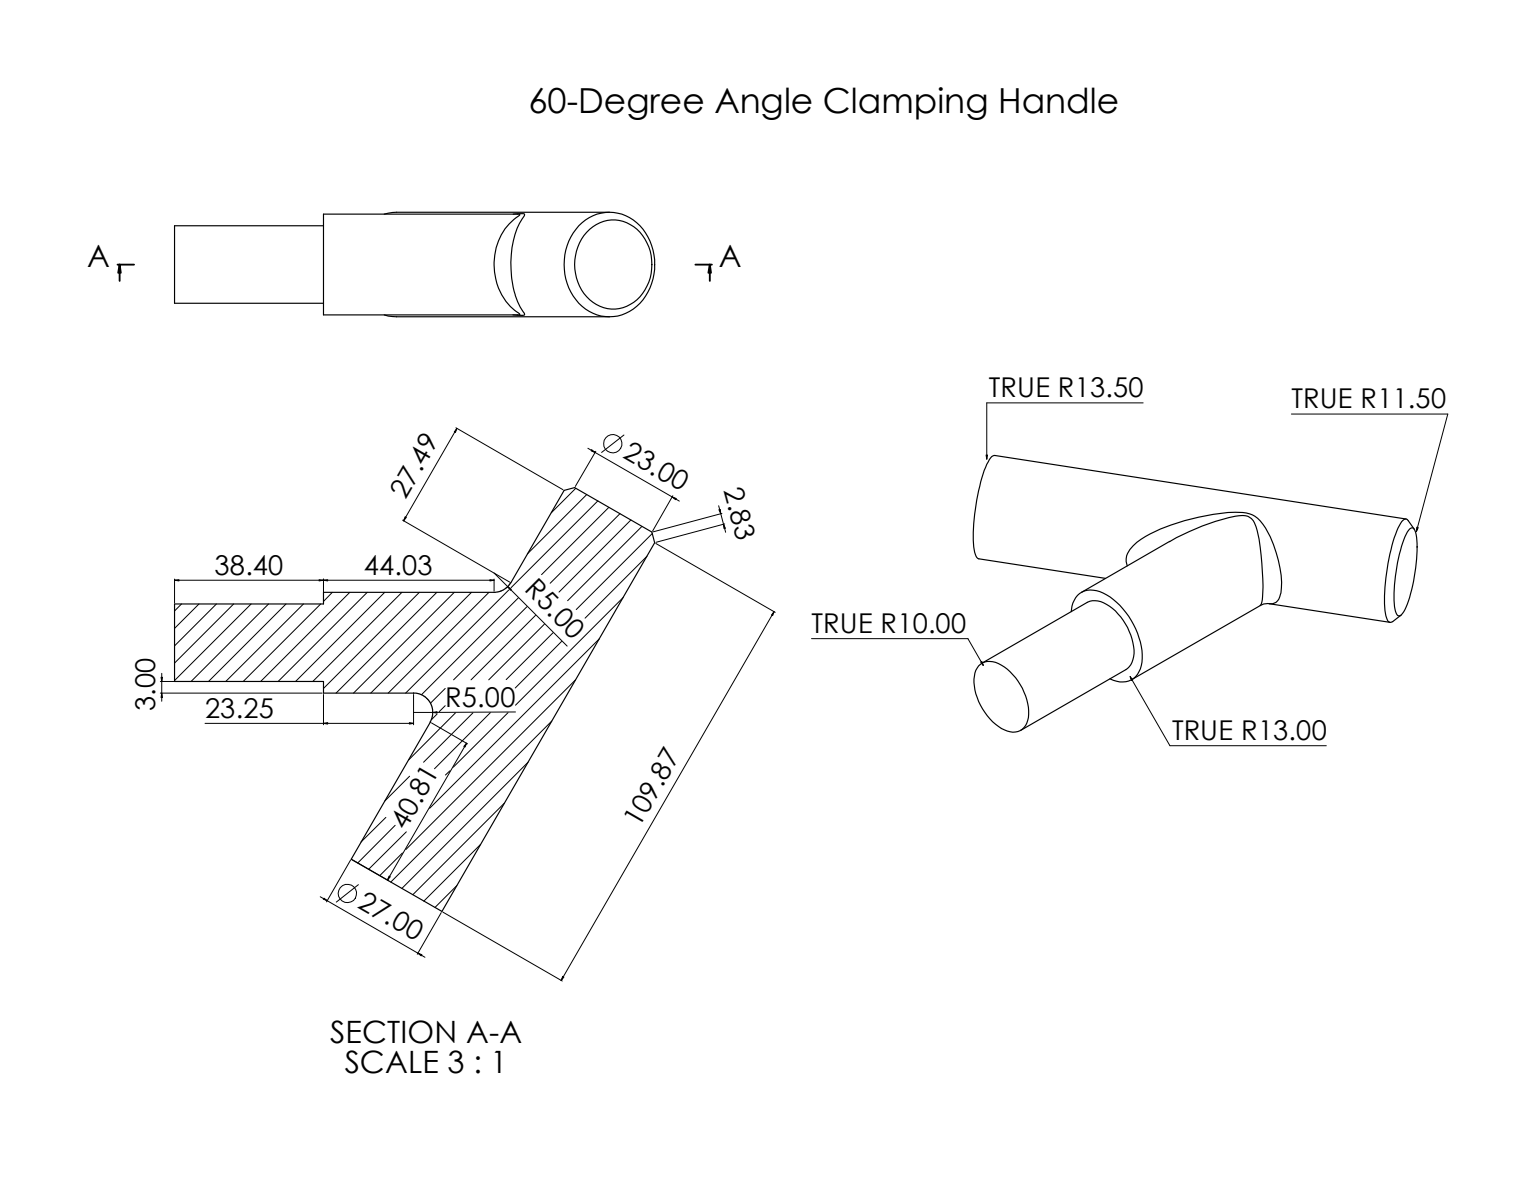
ISO-10303-21;
HEADER;
FILE_DESCRIPTION (('STEP AP214'),
    '1' );
FILE_NAME ('60-Degree Angle Clamping Handle.step',
    '2026-10-26T22:46:44',
    ( '' ),
    ( '' ),
    'SwSTEP 2.0',
    'SolidWorks 2025',
    '' );
FILE_SCHEMA (( 'AUTOMOTIVE_DESIGN' ));
ENDSEC;

DATA;
#3=CARTESIAN_POINT ( 'NONE',  ( 65.59213978856993776, 73.13321318536134186, -22.65145034150330616 ) ) ;
#7=CARTESIAN_POINT ( 'NONE',  ( 63.07699891084844523, 77.89006876494195808, -8.475025019650114899 ) ) ;
#33=CARTESIAN_POINT ( 'NONE',  ( 72.20123527641440830, 74.90140838070377072, -0.9291223156572469000 ) ) ;
#36=EDGE_CURVE ( 'NONE', #14580, #7029, #1544, .T. ) ;
#50=CARTESIAN_POINT ( 'NONE',  ( 54.22345804136912051, 78.00945976696758066, -12.46744236580036791 ) ) ;
#59=AXIS2_PLACEMENT_3D ( 'NONE', #20205, #816, #18936 ) ;
#61=EDGE_CURVE ( 'NONE', #19064, #20850, #19152, .T. ) ;
#66=B_SPLINE_CURVE_WITH_KNOTS ( 'NONE', 3,
 ( #8841, #10417, #10308, #18497, #16902, #3750, #6925, #16700, #20081, #8735, #685, #15341, #16481, #1963, #8630, #5225, #15026, #3643, #15129, #584, #2382, #3544, #11613, #795, #7034, #9988, #7140, #8411, #10096, #5431, #7246, #2073, #5545, #13520, #19652, #19965, #12034, #14912, #20596, #12135, #15751, #14164, #15438, #7666 ),
 .UNSPECIFIED., .F., .F.,
 ( 4, 2, 2, 2, 2, 2, 2, 2, 2, 2, 2, 2, 2, 2, 2, 2, 2, 2, 2, 2, 2, 4 ),
 ( 0.09617483233575800650, 0.09914136407045009980, 0.1006246299377961534, 0.1021078958051422070, 0.1050744275398343142, 0.1080409592745264352, 0.1095242251418725027, 0.1110074910092185702, 0.1139740227439106635, 0.1154572886112567032, 0.1169405544786027568, 0.1176821874122757766, 0.1184238203459488104, 0.1199070862132948084, 0.1213903520806408065, 0.1228736179479868185, 0.1258401496826788146, 0.1288066814173708385, 0.1317732131520628625, 0.1377062766214468548, 0.1406728083561389064, 0.1436393400908309581 ),
 .UNSPECIFIED. ) ;
#114=CARTESIAN_POINT ( 'NONE',  ( 60.67510459333478678, 75.25732190833497270, -4.504626686252581891 ) ) ;
#134=CARTESIAN_POINT ( 'NONE',  ( 79.71489363099678371, 68.48589378271981332, 0.4850882486192328313 ) ) ;
#137=CARTESIAN_POINT ( 'NONE',  ( 78.24291704612552678, 52.61578353862905288, -16.49051273642769289 ) ) ;
#149=CARTESIAN_POINT ( 'NONE',  ( 55.21771490548105987, 77.58705400462579860, -9.223793769219156502 ) ) ;
#167=CARTESIAN_POINT ( 'NONE',  ( 64.57205371728791476, 77.00255147951500589, -18.47244162738281048 ) ) ;
#187=CARTESIAN_POINT ( 'NONE',  ( 31.00000000000000711, 65.00000000000000000, 0.4999999999999970024 ) ) ;
#188=CARTESIAN_POINT ( 'NONE',  ( 61.55523633728010680, 134.3395726428436774, -12.50000000000000000 ) ) ;
#207=CARTESIAN_POINT ( 'NONE',  ( 54.88115708448756891, 77.73008567377026168, -9.852707893755395574 ) ) ;
#225=CARTESIAN_POINT ( 'NONE',  ( 58.57586221349340860, 85.49999999999941735, -12.75852093573072032 ) ) ;
#232=ORIENTED_EDGE ( 'NONE', *, *, #19491, .T. ) ;
#235=CARTESIAN_POINT ( 'NONE',  ( 82.91273300024698756, 62.96352848655696732, 0.4857625843512909936 ) ) ;
#237=CARTESIAN_POINT ( 'NONE',  ( 79.37077236198800279, 49.52807498578272316, -11.55216451523023657 ) ) ;
#250=CARTESIAN_POINT ( 'NONE',  ( 69.27805541368826425, 71.51676853726520733, -1.217222206000668994 ) ) ;
#268=CARTESIAN_POINT ( 'NONE',  ( 79.94330251453826008, 67.07585766759784462, -25.35419664930641659 ) ) ;
#308=CARTESIAN_POINT ( 'NONE',  ( 57.74218117268578965, 76.51201622986452833, -6.446212979376384489 ) ) ;
#332=VECTOR ( 'NONE', #6843, 1000.000000000000114 ) ;
#342=CARTESIAN_POINT ( 'NONE',  ( 76.94659547200038219, 54.56764967722406823, -20.27289619944112786 ) ) ;
#354=CARTESIAN_POINT ( 'NONE',  ( 76.60035650392514128, 54.09786888454211606, -5.411621923353880703 ) ) ;
#364=CARTESIAN_POINT ( 'NONE',  ( 54.28616200159638083, 77.98283342922744055, -13.21260929400889950 ) ) ;
#383=CARTESIAN_POINT ( 'NONE',  ( 81.91557740337785276, 60.53556548035048479, -24.72568746032316511 ) ) ;
#424=CARTESIAN_POINT ( 'NONE',  ( 64.92628429094538944, 80.60227088397526529, -21.04771496906974804 ) ) ;
#444=CARTESIAN_POINT ( 'NONE',  ( 116.4887320753796587, 39.19196698708793747, -12.50000000000000000 ) ) ;
#452=CARTESIAN_POINT ( 'NONE',  ( 77.98814704359870120, 52.13394603002385708, -14.43366844821333572 ) ) ;
#460=CARTESIAN_POINT ( 'NONE',  ( 76.86601529753625073, 54.45829969532270809, -4.885926103426701417 ) ) ;
#468=CARTESIAN_POINT ( 'NONE',  ( 58.42188568717646291, 76.22201287237797374, -19.09002448919735428 ) ) ;
#490=EDGE_CURVE ( 'NONE', #14308, #10603, #66, .T. ) ;
#492=CARTESIAN_POINT ( 'NONE',  ( 82.72938175528729232, 60.17526287326926848, -24.94610863806802925 ) ) ;
#510=CARTESIAN_POINT ( 'NONE',  ( 78.47145885649602803, 56.68941013563004816, -2.495457786690434610 ) ) ;
#516=EDGE_LOOP ( 'NONE', ( #16773, #17609, #13168, #2183, #18368 ) ) ;
#526=CARTESIAN_POINT ( 'NONE',  ( 54.80454468582367866, 77.76263990853003349, -14.98572519218623889 ) ) ;
#549=CARTESIAN_POINT ( 'NONE',  ( 82.83076346201933404, 60.85614612423834302, 0.1131946898860237832 ) ) ;
#551=CARTESIAN_POINT ( 'NONE',  ( 79.48072094348276551, 49.82842808374601162, -15.22942965609466270 ) ) ;
#584=CARTESIAN_POINT ( 'NONE',  ( 82.93056326137615031, 61.76632323605970498, -25.30877389655469756 ) ) ;
#588=CARTESIAN_POINT ( 'NONE',  ( 81.35624441458497813, 64.60845994063853936, -25.49655522582468237 ) ) ;
#594=CARTESIAN_POINT ( 'NONE',  ( 86.00000000000000000, 65.00000000000000000, -12.50000000000000000 ) ) ;
#609=CARTESIAN_POINT ( 'NONE',  ( 78.05328906524978549, 56.09831538232894843, -3.025823995327162841 ) ) ;
#628=CARTESIAN_POINT ( 'NONE',  ( 55.63769925775388714, 77.40847683933932899, -16.40349017008347587 ) ) ;
#651=CARTESIAN_POINT ( 'NONE',  ( 79.92501236954103661, 58.85901869437554268, -1.031643761997860897 ) ) ;
#660=CARTESIAN_POINT ( 'NONE',  ( 75.12482142704125465, 52.12498453794043485, -14.42445013263158238 ) ) ;
#685=CARTESIAN_POINT ( 'NONE',  ( 80.96866787924291486, 54.01966784746423400, -21.77093191989936471 ) ) ;
#687=DIRECTION ( 'NONE',  ( 0.8660254037844362651, 0.5000000000000043299, 0.000000000000000000 ) ) ;
#690=CARTESIAN_POINT ( 'NONE',  ( 80.82058163573867660, 65.29640235792498970, -25.49857619709358048 ) ) ;
#692=CARTESIAN_POINT ( 'NONE',  ( 59.45914026090133575, 84.82127241994479050, -15.89427485249682626 ) ) ;
#713=CARTESIAN_POINT ( 'NONE',  ( 79.12402306321216372, 57.63706906876117131, -1.778930141804763831 ) ) ;
#735=CARTESIAN_POINT ( 'NONE',  ( 60.75134160315762699, 83.82709006120157369, -17.71883169751006548 ) ) ;
#765=CARTESIAN_POINT ( 'NONE',  ( 81.28584910398754459, 61.36302568043885941, -0.01657068726255144647 ) ) ;
#773=CARTESIAN_POINT ( 'NONE',  ( 78.91362683933590461, 57.32445438350235634, -23.00962568793631036 ) ) ;
#779=MECHANICAL_DESIGN_GEOMETRIC_PRESENTATION_REPRESENTATION('',(#4502),#19384);
#795=CARTESIAN_POINT ( 'NONE',  ( 82.80106909841869367, 63.71549435008554241, -25.56184987062727743 ) ) ;
#800=CARTESIAN_POINT ( 'NONE',  ( 81.32899831459523909, 65.64633111285905898, -25.49135248455479541 ) ) ;
#816=DIRECTION ( 'NONE',  ( 1.000000000000000000, -0.000000000000000000, -0.000000000000000000 ) ) ;
#838=CARTESIAN_POINT ( 'NONE',  ( 63.10828723790488937, 82.00971617295591898, -19.89823807612492601 ) ) ;
#863=CARTESIAN_POINT ( 'NONE',  ( 81.25108741995337880, 54.86839436850289076, -2.588578014267536975 ) ) ;
#875=FACE_BOUND ( 'NONE', #4618, .T. ) ;
#955=DIRECTION ( 'NONE',  ( 0.5705585702127619063, 0.000000000000000000, 0.8212569134910030488 ) ) ;
#957=CARTESIAN_POINT ( 'NONE',  ( -7.400583024429460366, 65.00000000000000000, -12.50000000000000000 ) ) ;
#967=CARTESIAN_POINT ( 'NONE',  ( 80.52543256968870367, 57.14253470624510811, -2.115012055466068741 ) ) ;
#969=ORIENTED_EDGE ( 'NONE', *, *, #20916, .T. ) ;
#973=CARTESIAN_POINT ( 'NONE',  ( 79.14338724215045318, 54.34411555289009499, -5.006392671230091906 ) ) ;
#991=PLANE ( 'NONE',  #9815 ) ;
#1001=AXIS2_PLACEMENT_3D ( 'NONE', #3701, #10052, #11562 ) ;
#1027=CARTESIAN_POINT ( 'NONE',  ( 80.02281011973705915, 51.32424184041445159, -6.278812083988356996 ) ) ;
#1031=CONICAL_SURFACE ( 'NONE', #12883, 11.50000000000002309, 0.7853981633974477239 ) ;
#1052=ORIENTED_EDGE ( 'NONE', *, *, #9633, .T. ) ;
#1077=CARTESIAN_POINT ( 'NONE',  ( 75.33430881385784517, 70.41445892100490767, -0.5834797149646978598 ) ) ;
#1137=ORIENTED_EDGE ( 'NONE', *, *, #36, .F. ) ;
#1182=CARTESIAN_POINT ( 'NONE',  ( 76.96076175570429712, 69.31984913612060950, -0.1862401116020122038 ) ) ;
#1202=DIRECTION ( 'NONE',  ( -0.5000000000000045519, 0.8660254037844360431, 0.000000000000000000 ) ) ;
#1274=DIRECTION ( 'NONE',  ( 0.000000000000000000, 0.000000000000000000, 1.000000000000000000 ) ) ;
#1289=CARTESIAN_POINT ( 'NONE',  ( 71.98518577010987940, 75.06736630765306018, -1.005590943479974131 ) ) ;
#1309=CARTESIAN_POINT ( 'NONE',  ( -7.400583024429460366, 65.00000000000000000, -2.500000000000005773 ) ) ;
#1379=CARTESIAN_POINT ( 'NONE',  ( 61.57468973143931379, 74.87077495648827608, -20.95977551465544764 ) ) ;
#1387=CARTESIAN_POINT ( 'NONE',  ( 77.64194032647326082, 70.38417867298623776, 0.2137292797775141029 ) ) ;
#1409=EDGE_CURVE ( 'NONE', #2714, #10603, #16734, .T. ) ;
#1417=CARTESIAN_POINT ( 'NONE',  ( 58.59049733147158889, 85.48875911470162237, -11.99710087975904216 ) ) ;
#1456=CARTESIAN_POINT ( 'NONE',  ( 64.92628429094538944, 80.60227088397526529, -21.04771496906974448 ) ) ;
#1490=CARTESIAN_POINT ( 'NONE',  ( 82.46725602463313010, 64.79916592910645079, 0.6251661754290179784 ) ) ;
#1503=CARTESIAN_POINT ( 'NONE',  ( 86.00000000000000000, 65.00000000000000000, -12.50000000000000000 ) ) ;
#1518=CARTESIAN_POINT ( 'NONE',  ( 82.69314351557979137, 60.01919287894784105, -0.1021492064584022391 ) ) ;
#1544=CIRCLE ( 'NONE', #20817, 13.49999999999999645 ) ;
#1586=CARTESIAN_POINT ( 'NONE',  ( 68.05653244943854929, 72.05492144323341108, -23.45593384645862045 ) ) ;
#1591=PLANE ( 'NONE',  #12909 ) ;
#1595=CARTESIAN_POINT ( 'NONE',  ( 60.86250686525652753, 83.74154639049930893, -7.143441593098562414 ) ) ;
#1638=CARTESIAN_POINT ( 'NONE',  ( 79.60954748500523692, 66.31227659742221192, 0.4370474645863004493 ) ) ;
#1657=CARTESIAN_POINT ( 'NONE',  ( 75.15087072258846490, 70.53326157795075346, -24.36499220651786146 ) ) ;
#1659=CIRCLE ( 'NONE', #19280, 9.999999999999994671 ) ;
#1661=CARTESIAN_POINT ( 'NONE',  ( 105.7973891242897650, 30.70991617951901276, -12.50000000000000000 ) ) ;
#1694=CARTESIAN_POINT ( 'NONE',  ( 55.27961512323265225, 77.56072257029609318, -9.140361019020206257 ) ) ;
#1706=CARTESIAN_POINT ( 'NONE',  ( 31.00000000000000711, 65.00000000000000000, -12.50000000000000000 ) ) ;
#1719=CARTESIAN_POINT ( 'NONE',  ( 82.78189083499628964, 60.49709294355461253, 0.02860270449327129150 ) ) ;
#1725=CARTESIAN_POINT ( 'NONE',  ( 77.91922477836661187, 52.00401066416952034, -13.06454345700202424 ) ) ;
#1742=CARTESIAN_POINT ( 'NONE',  ( 57.02843452872113517, 76.81644352065700332, -7.029764943285477408 ) ) ;
#1762=CARTESIAN_POINT ( 'NONE',  ( 76.57684527313351452, 68.08025284203007743, -25.13374168853553670 ) ) ;
#1764=ADVANCED_FACE ( 'NONE', ( #10312 ), #15343, .T. ) ;
#1804=CARTESIAN_POINT ( 'NONE',  ( 62.19571619003149010, 78.41436756500478111, -11.69768420993622904 ) ) ;
#1824=CARTESIAN_POINT ( 'NONE',  ( 78.98475196968189493, 69.17512925677146995, 0.4016226566437379741 ) ) ;
#1829=CARTESIAN_POINT ( 'NONE',  ( 75.20419437876392976, 52.23006250689047647, -10.01053177166429542 ) ) ;
#1847=CARTESIAN_POINT ( 'NONE',  ( 56.65135822015081146, 76.97701555849656074, -17.56718000666989354 ) ) ;
#1865=CARTESIAN_POINT ( 'NONE',  ( 78.39368881307802894, 68.30389099123098617, -25.10803604556682700 ) ) ;
#1905=ORIENTED_EDGE ( 'NONE', *, *, #2268, .T. ) ;
#1908=CARTESIAN_POINT ( 'NONE',  ( 62.82311980245329153, 82.22968959821695023, -5.348578013552717003 ) ) ;
#1936=CARTESIAN_POINT ( 'NONE',  ( 79.67147709189563898, 50.35212617480907227, -8.215081154367272376 ) ) ;
#1940=ORIENTED_EDGE ( 'NONE', *, *, #10019, .F. ) ;
#1950=CARTESIAN_POINT ( 'NONE',  ( 71.88466637961029448, 70.33575297470315491, -0.6373663580885260416 ) ) ;
#1951=VECTOR ( 'NONE', #13576, 1000.000000000000000 ) ;
#1961=DIRECTION ( 'NONE',  ( 1.000000000000000000, -0.000000000000000000, -0.000000000000000000 ) ) ;
#1963=CARTESIAN_POINT ( 'NONE',  ( 81.73016281821475104, 56.36132269136237483, -23.36898426428367870 ) ) ;
#1969=CARTESIAN_POINT ( 'NONE',  ( 68.88680438096986336, 74.41951537632650115, -21.80366467887538917 ) ) ;
#1975=DIRECTION ( 'NONE',  ( 0.5000000000000044409, -0.8660254037844361541, 0.000000000000000000 ) ) ;
#2008=CARTESIAN_POINT ( 'NONE',  ( 59.23362366115814837, 84.99461582490647515, -9.581601599933526003 ) ) ;
#2010=CIRCLE ( 'NONE', #1001, 13.50000000000000178 ) ;
#2038=CARTESIAN_POINT ( 'NONE',  ( 78.11286510409185269, 52.36951057819560873, -9.387962703321013791 ) ) ;
#2047=CARTESIAN_POINT ( 'NONE',  ( 79.92771531775157712, 58.85638066918279065, -23.97260934375448471 ) ) ;
#2055=CARTESIAN_POINT ( 'NONE',  ( 75.36551866217324402, 68.69483139169550157, -0.02780010607275849518 ) ) ;
#2069=DIRECTION ( 'NONE',  ( 0.000000000000000000, 0.000000000000000000, -1.000000000000000000 ) ) ;
#2073=CARTESIAN_POINT ( 'NONE',  ( 79.61145830677504875, 68.58534652329807102, -25.47370545880939474 ) ) ;
#2079=CARTESIAN_POINT ( 'NONE',  ( 81.66920570542281155, 63.84695342301056797, -25.45140023156622533 ) ) ;
#2111=CONICAL_SURFACE ( 'NONE', #13969, 11.50000000000002309, 0.7853981633974477239 ) ;
#2120=CARTESIAN_POINT ( 'NONE',  ( 60.24514846279297586, 84.21671670512185415, -17.09502645871620885 ) ) ;
#2144=CARTESIAN_POINT ( 'NONE',  ( 82.25469362684589214, 61.96434487962967808, 0.1446237860341569037 ) ) ;
#2147=CARTESIAN_POINT ( 'NONE',  ( 78.60734359744111543, 53.30791790663061391, -6.696939495182443025 ) ) ;
#2155=CARTESIAN_POINT ( 'NONE',  ( 77.73754876681609005, 55.65438722760616486, -3.442927121160782367 ) ) ;
#2183=ORIENTED_EDGE ( 'NONE', *, *, #17676, .T. ) ;
#2184=CARTESIAN_POINT ( 'NONE',  ( 81.90911831446538827, 56.94440004289425872, -23.68671869826702547 ) ) ;
#2219=CARTESIAN_POINT ( 'NONE',  ( 58.57279107162051446, 85.50235892223300027, -12.67366829707468057 ) ) ;
#2246=CARTESIAN_POINT ( 'NONE',  ( 78.30707807390135144, 56.45514055384987984, -2.690560523447495633 ) ) ;
#2249=CARTESIAN_POINT ( 'NONE',  ( 77.08812400714005264, 54.76052789366846696, -4.475059266215096088 ) ) ;
#2266=CARTESIAN_POINT ( 'NONE',  ( -7.400583024429460366, 65.00000000000000000, -12.50000000000000000 ) ) ;
#2268=EDGE_CURVE ( 'NONE', #13099, #5375, #13227, .T. ) ;
#2285=CARTESIAN_POINT ( 'NONE',  ( 82.33150071157334082, 63.03942819492690575, -25.35471444149103348 ) ) ;
#2326=CARTESIAN_POINT ( 'NONE',  ( 59.78152309849413371, 84.57340574088013341, -16.44406699097515911 ) ) ;
#2350=FACE_OUTER_BOUND ( 'NONE', #11102, .T. ) ;
#2353=CARTESIAN_POINT ( 'NONE',  ( 80.96203380818354844, 54.00641746404563293, -3.266085604399942000 ) ) ;
#2359=CARTESIAN_POINT ( 'NONE',  ( 80.58279200417960908, 59.94663314240338536, -24.49284399293752301 ) ) ;
#2382=CARTESIAN_POINT ( 'NONE',  ( 82.95222531821094947, 62.25068779409587449, -25.39145899207881030 ) ) ;
#2387=CARTESIAN_POINT ( 'NONE',  ( 81.35960895894935163, 61.54332286617361802, -25.03457989382592430 ) ) ;
#2389=CARTESIAN_POINT ( 'NONE',  ( 64.18815039242018372, 81.17459403355988456, -20.61608748715355333 ) ) ;
#2431=CARTESIAN_POINT ( 'NONE',  ( 58.88264075909191320, 85.26433268085669681, -14.50872457446225461 ) ) ;
#2464=CARTESIAN_POINT ( 'NONE',  ( 79.78989234911249184, 55.62452637193754867, -3.470983589548607640 ) ) ;
#2518=CARTESIAN_POINT ( 'NONE',  ( 81.39009893423684616, 61.60396693986834293, 0.05555408759164950916 ) ) ;
#2538=CARTESIAN_POINT ( 'NONE',  ( 63.99383217623863374, 81.32526156698924069, -20.50245894047660755 ) ) ;
#2573=EDGE_CURVE ( 'NONE', #8298, #5808, #6631, .T. ) ;
#2625=CARTESIAN_POINT ( 'NONE',  ( 81.10655718899290889, 54.43739570252013493, -2.927339837283823520 ) ) ;
#2654=DIRECTION ( 'NONE',  ( -0.9659258262890694224, 0.2588190451025162431, 0.000000000000000000 ) ) ;
#2668=CARTESIAN_POINT ( 'NONE',  ( 73.24173739811655537, 69.71069241403367300, -0.3690567165748998568 ) ) ;
#2684=EDGE_CURVE ( 'NONE', #3901, #12877, #16827, .T. ) ;
#2714=VERTEX_POINT ( 'NONE', #13652 ) ;
#2724=EDGE_LOOP ( 'NONE', ( #9285, #1905 ) ) ;
#2774=CARTESIAN_POINT ( 'NONE',  ( 81.47405289336727208, 65.45330303017013307, 0.4987988714753746611 ) ) ;
#2816=EDGE_CURVE ( 'NONE', #20850, #14308, #9590, .T. ) ;
#2830=EDGE_CURVE ( 'NONE', #8298, #11548, #12930, .T. ) ;
#2832=CARTESIAN_POINT ( 'NONE',  ( 80.63605647399829479, 53.05720336860252928, -4.117601259720633955 ) ) ;
#2867=CARTESIAN_POINT ( 'NONE',  ( 74.06428810979899424, 71.22525070374874190, -24.03620132832545764 ) ) ;
#2876=CARTESIAN_POINT ( 'NONE',  ( 73.00847438502604803, 74.24912532398991516, -0.7262419208828606587 ) ) ;
#2979=CARTESIAN_POINT ( 'NONE',  ( 71.09010947823266235, 73.07777849309526630, -2.093657812535054674 ) ) ;
#3003=CARTESIAN_POINT ( 'NONE',  ( 58.57586221349259858, 85.50000000000002842, -12.50000000002017231 ) ) ;
#3036=CARTESIAN_POINT ( 'NONE',  ( -7.400583024429460366, 65.00000000000000000, -22.49999999999999645 ) ) ;
#3071=CARTESIAN_POINT ( 'NONE',  ( 79.27926581092380331, 66.53148362518940928, -25.41189871557945068 ) ) ;
#3080=CARTESIAN_POINT ( 'NONE',  ( 81.73881534337073163, 63.13855879245894442, 0.3687221123209319384 ) ) ;
#3110=CARTESIAN_POINT ( 'NONE',  ( 82.31088920383102447, 65.12868601141531144, 0.6320188806532470727 ) ) ;
#3142=EDGE_CURVE ( 'NONE', #5200, #12877, #18673, .T. ) ;
#3181=CARTESIAN_POINT ( 'NONE',  ( 63.25496377350514621, 81.89610108269177147, -5.027972649527582938 ) ) ;
#3227=AXIS2_PLACEMENT_3D ( 'NONE', #10123, #16928, #12061 ) ;
#3230=CIRCLE ( 'NONE', #5242, 12.99999999999999822 ) ;
#3279=CARTESIAN_POINT ( 'NONE',  ( 60.03527469150965601, 84.37819276222457177, -8.194308862602044385 ) ) ;
#3309=CARTESIAN_POINT ( 'NONE',  ( 81.95753769289619584, 65.79275367316732570, 0.6382041694687864419 ) ) ;
#3312=CARTESIAN_POINT ( 'NONE',  ( 78.01023140970075076, 52.17558613751951668, -10.30093800761554412 ) ) ;
#3329=CARTESIAN_POINT ( 'NONE',  ( 61.62883818700242955, 74.84782268386872772, -3.995215303412941399 ) ) ;
#3345=CARTESIAN_POINT ( 'NONE',  ( 79.00508257797014267, 69.14961577860513842, -25.40092402025251062 ) ) ;
#3377=CARTESIAN_POINT ( 'NONE',  ( 61.99846457528121135, 82.86613150643367476, -6.025952610566521095 ) ) ;
#3389=CYLINDRICAL_SURFACE ( 'NONE', #9093, 12.99999999999999822 ) ;
#3395=CARTESIAN_POINT ( 'NONE',  ( 58.57586221349259858, 85.50000000000002842, -12.50000000002017231 ) ) ;
#3404=CARTESIAN_POINT ( 'NONE',  ( 60.45545169401432162, 84.05486846333056405, -7.636015506719354917 ) ) ;
#3409=CARTESIAN_POINT ( 'NONE',  ( 75.06184213092844004, 52.04164024659630172, -13.66203483571357147 ) ) ;
#3428=CARTESIAN_POINT ( 'NONE',  ( 54.97757980634291641, 77.68911581231870400, -9.638134293611450687 ) ) ;
#3443=AXIS2_PLACEMENT_3D ( 'NONE', #15840, #7658, #20700 ) ;
#3448=CARTESIAN_POINT ( 'NONE',  ( 79.50714813094847955, 68.67338619406606881, -25.45940246541340457 ) ) ;
#3491=CARTESIAN_POINT ( 'NONE',  ( 55.43008045110529025, 77.49674724409801740, -8.910180418637997590 ) ) ;
#3516=CARTESIAN_POINT ( 'NONE',  ( 79.56990498979357085, 50.07294208995298135, -8.967104414842829385 ) ) ;
#3530=CARTESIAN_POINT ( 'NONE',  ( 74.49564010550007254, 69.11503523615289168, -0.1607087966260463130 ) ) ;
#3544=CARTESIAN_POINT ( 'NONE',  ( 82.91030674320427352, 62.98464439186960107, -25.48828433254854176 ) ) ;
#3549=CARTESIAN_POINT ( 'NONE',  ( 75.99050373817134130, 68.37836398556720496, -25.05701615029671459 ) ) ;
#3565=CARTESIAN_POINT ( 'NONE',  ( 31.00000000000000711, 65.00000000000000000, -12.50000000000000000 ) ) ;
#3567=ORIENTED_EDGE ( 'NONE', *, *, #16034, .T. ) ;
#3589=CARTESIAN_POINT ( 'NONE',  ( 59.88327620991913847, 84.49511162386195906, -8.417773832668045131 ) ) ;
#3615=CARTESIAN_POINT ( 'NONE',  ( 75.13664552285537468, 52.14064219013824442, -10.52251561064948682 ) ) ;
#3643=CARTESIAN_POINT ( 'NONE',  ( 82.75100189971391274, 60.33120646178909396, -24.98450340712203044 ) ) ;
#3649=CARTESIAN_POINT ( 'NONE',  ( 82.19612864528707519, 65.36250969618502893, -25.63618266340674978 ) ) ;
#3667=CARTESIAN_POINT ( 'NONE',  ( 79.78236940327508364, 58.62749654732350280, -1.141850372723110629 ) ) ;
#3677=DIRECTION ( 'NONE',  ( 0.8660254037844362651, 0.5000000000000043299, 0.000000000000000000 ) ) ;
#3685=CARTESIAN_POINT ( 'NONE',  ( 62.90924860651898598, 77.99809401039773604, -12.47726437862388948 ) ) ;
#3701=CARTESIAN_POINT ( 'NONE',  ( 49.86389338619021316, 127.5895726428436205, -12.50000000000000000 ) ) ;
#3716=CARTESIAN_POINT ( 'NONE',  ( 75.96605662148094495, 53.24384717281555623, -18.14283704812129017 ) ) ;
#3725=CARTESIAN_POINT ( 'NONE',  ( 81.72727647338570023, 63.41126555804013520, -25.40372688915182664 ) ) ;
#3750=CARTESIAN_POINT ( 'NONE',  ( 79.74209024524658673, 50.54664088538957856, -17.24859437997715972 ) ) ;
#3760=CARTESIAN_POINT ( 'NONE',  ( 81.86472787884530078, 64.82771547793723244, -25.50399698552627115 ) ) ;
#3768=ADVANCED_FACE ( 'NONE', ( #12344 ), #991, .T. ) ;
#3779=CARTESIAN_POINT ( 'NONE',  ( 81.62020900107658861, 64.01414927466113625, 0.4645082096952444228 ) ) ;
#3790=CYLINDRICAL_SURFACE ( 'NONE', #17013, 13.50000000000000711 ) ;
#3798=CARTESIAN_POINT ( 'NONE',  ( 62.27440062445415947, 78.36885602720158772, -12.89736757990179861 ) ) ;
#3835=CARTESIAN_POINT ( 'NONE',  ( 76.02931450606715202, 53.32891420438221530, -18.26399853987619792 ) ) ;
#3841=EDGE_CURVE ( 'NONE', #13156, #6779, #18587, .T. ) ;
#3865=CARTESIAN_POINT ( 'NONE',  ( 80.87396291321206832, 53.74885471499349876, -21.51050425557589918 ) ) ;
#3881=ORIENTED_EDGE ( 'NONE', *, *, #19491, .F. ) ;
#3901=VERTEX_POINT ( 'NONE', #1309 ) ;
#3902=CARTESIAN_POINT ( 'NONE',  ( 58.80800210575738163, 85.32167585634152829, -14.25381645728047708 ) ) ;
#3929=ADVANCED_FACE ( 'NONE', ( #18908 ), #1031, .T. ) ;
#3933=CARTESIAN_POINT ( 'NONE',  ( 82.14679489777772403, 61.41165722483968636, -0.0001489139912725718411 ) ) ;
#3943=CARTESIAN_POINT ( 'NONE',  ( 81.73281949542425195, 63.23532430020726025, -25.38086878997933837 ) ) ;
#3975=CARTESIAN_POINT ( 'NONE',  ( 80.79037351930210775, 57.71461494556285743, -23.29247368251557759 ) ) ;
#3998=CARTESIAN_POINT ( 'NONE',  ( 104.7973891242897650, 32.44196698708787352, -12.50000000000000000 ) ) ;
#4010=CARTESIAN_POINT ( 'NONE',  ( 62.57915299879362436, 78.18516598039407484, -15.53707111529713636 ) ) ;
#4033=CARTESIAN_POINT ( 'NONE',  ( 81.70299675858660748, 56.27235011262846598, -1.678517931375763883 ) ) ;
#4042=CARTESIAN_POINT ( 'NONE',  ( 81.17621279504307097, 64.86352945118836999, -25.50000000000000355 ) ) ;
#4074=AXIS2_PLACEMENT_3D ( 'NONE', #594, #16811, #16491 ) ;
#4078=CARTESIAN_POINT ( 'NONE',  ( 81.37385535124417402, 59.06361191445762415, -24.08546180346211685 ) ) ;
#4084=CYLINDRICAL_SURFACE ( 'NONE', #4074, 12.99999999999999822 ) ;
#4093=DIRECTION ( 'NONE',  ( 0.000000000000000000, 0.000000000000000000, -1.000000000000000000 ) ) ;
#4121=CARTESIAN_POINT ( 'NONE',  ( 62.43702563953799967, 78.27403789581164517, -12.60076481416450989 ) ) ;
#4149=CARTESIAN_POINT ( 'NONE',  ( 82.15152675072569366, 57.78258148490818513, -0.9124300798289324277 ) ) ;
#4195=ADVANCED_FACE ( 'NONE', ( #2350 ), #11504, .F. ) ;
#4223=ORIENTED_EDGE ( 'NONE', *, *, #1409, .F. ) ;
#4250=DIRECTION ( 'NONE',  ( 0.5000000000000044409, -0.8660254037844361541, 0.000000000000000000 ) ) ;
#4253=CARTESIAN_POINT ( 'NONE',  ( 76.09784680959502623, 71.72003589649941091, -0.03901844198412815490 ) ) ;
#4259=CARTESIAN_POINT ( 'NONE',  ( 79.61537190921880836, 55.27319793895139100, -3.834855963081625241 ) ) ;
#4328=CARTESIAN_POINT ( 'NONE',  ( -7.400583024429460366, 65.00000000000000000, -12.50000000000000000 ) ) ;
#4356=CARTESIAN_POINT ( 'NONE',  ( 81.76460255947399958, 66.07321026818675591, 0.6318735725429163175 ) ) ;
#4424=CYLINDRICAL_SURFACE ( 'NONE', #5728, 9.999999999999994671 ) ;
#4428=ORIENTED_EDGE ( 'NONE', *, *, #61, .F. ) ;
#4451=DIRECTION ( 'NONE',  ( 0.000000000000000000, 0.000000000000000000, -1.000000000000000000 ) ) ;
#4452=CARTESIAN_POINT ( 'NONE',  ( 80.48184134440170112, 67.67503062758028420, -25.55523453281406887 ) ) ;
#4464=CARTESIAN_POINT ( 'NONE',  ( 72.13472612272360607, 72.43562250713796402, -1.655863322246043268 ) ) ;
#4502=STYLED_ITEM('',(#20974),#10712);
#4546=ORIENTED_EDGE ( 'NONE', *, *, #16748, .T. ) ;
#4555=CARTESIAN_POINT ( 'NONE',  ( 71.78648230981508505, 75.22576515165123112, -23.93658930654907380 ) ) ;
#4565=CARTESIAN_POINT ( 'NONE',  ( 78.57212408006208193, 68.17132923325316085, 0.1403190541435616057 ) ) ;
#4618=EDGE_LOOP ( 'NONE', ( #20810, #14203 ) ) ;
#4632=EDGE_CURVE ( 'NONE', #12877, #5200, #7093, .T. ) ;
#4663=CARTESIAN_POINT ( 'NONE',  ( 81.71790390665692883, 62.87457526787128614, 0.3277555819696695849 ) ) ;
#4673=EDGE_LOOP ( 'NONE', ( #5151, #12437 ) ) ;
#4676=DIRECTION ( 'NONE',  ( 0.000000000000000000, 0.000000000000000000, 1.000000000000000000 ) ) ;
#4689=CARTESIAN_POINT ( 'NONE',  ( 82.94492693169769382, 61.96459963853332198, 0.3444023811076172281 ) ) ;
#4728=DIRECTION ( 'NONE',  ( 0.5000000000000041078, -0.8660254037844362651, 0.000000000000000000 ) ) ;
#4756=CARTESIAN_POINT ( 'NONE',  ( 74.76692331049709139, 68.98407507634522062, -24.88169789286644118 ) ) ;
#4764=CARTESIAN_POINT ( 'NONE',  ( 54.41450017449287913, 77.92833245222763594, -11.11271623845599699 ) ) ;
#4871=CARTESIAN_POINT ( 'NONE',  ( 56.48324548572979609, 77.04861762647422552, -7.597113510449146290 ) ) ;
#4885=FACE_OUTER_BOUND ( 'NONE', #516, .T. ) ;
#4897=CARTESIAN_POINT ( 'NONE',  ( 59.03558430264390466, 85.14681185468893432, -10.05295229902272425 ) ) ;
#4899=CARTESIAN_POINT ( 'NONE',  ( 80.10952826493171131, 51.56390520361809138, -19.09971892243163438 ) ) ;
#4928=CARTESIAN_POINT ( 'NONE',  ( 77.72754490146294870, 67.46424320799033580, -25.26819846475408227 ) ) ;
#4946=ORIENTED_EDGE ( 'NONE', *, *, #2830, .T. ) ;
#4967=CARTESIAN_POINT ( 'NONE',  ( 59.47135335676293977, 84.81187091046737692, -9.105437536888221217 ) ) ;
#4990=CARTESIAN_POINT ( 'NONE',  ( 58.64832549623106672, 85.44433982373099923, -11.49787480049970334 ) ) ;
#4993=CARTESIAN_POINT ( 'NONE',  ( 78.65134511289586783, 53.39203929102664858, -18.47032050442678397 ) ) ;
#5029=CARTESIAN_POINT ( 'NONE',  ( 71.93434708225751706, 72.55958424763308301, -23.26416705100350768 ) ) ;
#5048=DIRECTION ( 'NONE',  ( 1.000000000000000000, -0.000000000000000000, -0.000000000000000000 ) ) ;
#5068=CARTESIAN_POINT ( 'NONE',  ( 62.81266095603159272, 74.33819947169733666, -3.428479281352090347 ) ) ;
#5093=CARTESIAN_POINT ( 'NONE',  ( 63.30970132782791637, 81.85394346738576132, -4.971994580379090145 ) ) ;
#5096=CARTESIAN_POINT ( 'NONE',  ( 75.33920648802740061, 52.40915241012807968, -9.253810560353768366 ) ) ;
#5114=CARTESIAN_POINT ( 'NONE',  ( 54.49397420869091491, 77.89457764545490193, -14.16833317594359798 ) ) ;
#5133=CARTESIAN_POINT ( 'NONE',  ( 73.03466427698670316, 69.80725080074495281, -24.59324696420904033 ) ) ;
#5151=ORIENTED_EDGE ( 'NONE', *, *, #2830, .F. ) ;
#5169=CARTESIAN_POINT ( 'NONE',  ( 62.23039322790586425, 78.39221673943322344, -10.60002489424368122 ) ) ;
#5196=CARTESIAN_POINT ( 'NONE',  ( 80.47222577874747174, 52.59073085207923270, -20.35369553621190519 ) ) ;
#5200=VERTEX_POINT ( 'NONE', #12946 ) ;
#5204=CARTESIAN_POINT ( 'NONE',  ( 75.64423735160997353, 52.81473335711799422, -17.04225810597251467 ) ) ;
#5212=CARTESIAN_POINT ( 'NONE',  ( 56.06633208239072985, 77.22609791612467234, -8.065985790676100109 ) ) ;
#5225=CARTESIAN_POINT ( 'NONE',  ( 82.23375342391803144, 58.06063708979128535, -24.22722688745409769 ) ) ;
#5230=CARTESIAN_POINT ( 'NONE',  ( 80.29132060388693048, 59.45028869689328133, -24.26604442088980917 ) ) ;
#5242=AXIS2_PLACEMENT_3D ( 'NONE', #1706, #8155, #14667 ) ;
#5273=CARTESIAN_POINT ( 'NONE',  ( 58.67095626531940411, 85.42695601701730368, -11.35807125314311072 ) ) ;
#5297=CARTESIAN_POINT ( 'NONE',  ( 77.91539758371193614, 51.99679936220445597, -12.14267250949680488 ) ) ;
#5305=CARTESIAN_POINT ( 'NONE',  ( 75.40630481554458697, 52.49822515946223689, -16.08063866060412650 ) ) ;
#5333=CARTESIAN_POINT ( 'NONE',  ( 82.31640018076895160, 62.45399354285202520, -25.25199697837627255 ) ) ;
#5336=FACE_OUTER_BOUND ( 'NONE', #16621, .T. ) ;
#5353=CARTESIAN_POINT ( 'NONE',  ( 81.03699745905494467, 60.80382008804202343, -0.1887428286780195308 ) ) ;
#5374=CARTESIAN_POINT ( 'NONE',  ( 62.89558499432746430, 78.00608458378800947, -12.44082293186782628 ) ) ;
#5375=VERTEX_POINT ( 'NONE', #20227 ) ;
#5400=CARTESIAN_POINT ( 'NONE',  ( 80.95969170222095102, 60.64095424398406919, -0.2422237528172087040 ) ) ;
#5402=CARTESIAN_POINT ( 'NONE',  ( 80.55381169140011366, 52.82318510880671170, -4.391639923843643878 ) ) ;
#5411=CARTESIAN_POINT ( 'NONE',  ( 75.89995346768556317, 53.15581343745467535, -7.100154262375115266 ) ) ;
#5431=CARTESIAN_POINT ( 'NONE',  ( 80.94022347753882229, 67.15523189662422965, -25.58958341134216852 ) ) ;
#5438=CARTESIAN_POINT ( 'NONE',  ( 81.73869807597520776, 63.32742336881895540, -25.39460242813820656 ) ) ;
#5439=CARTESIAN_POINT ( 'NONE',  ( 61.44066546377918314, 83.29626644201148622, -18.49058275380094685 ) ) ;
#5458=CARTESIAN_POINT ( 'NONE',  ( 81.06711713768373784, 65.00000000000000000, 0.4999999999999962252 ) ) ;
#5460=DIRECTION ( 'NONE',  ( 0.8660254037844358210, 0.5000000000000046629, 0.000000000000000000 ) ) ;
#5482=CARTESIAN_POINT ( 'NONE',  ( 58.60004645507417820, 85.48142452582160900, -11.88094507543154421 ) ) ;
#5504=ORIENTED_EDGE ( 'NONE', *, *, #2268, .F. ) ;
#5522=CARTESIAN_POINT ( 'NONE',  ( 81.70617321326079718, 62.71419586981366479, -25.30228666757756528 ) ) ;
#5545=CARTESIAN_POINT ( 'NONE',  ( 78.90035330931522140, 69.25335659932615329, -25.39095082874599285 ) ) ;
#5549=CARTESIAN_POINT ( 'NONE',  ( 81.75619180876375935, 56.44393855648663560, -23.41859921127574395 ) ) ;
#5550=CARTESIAN_POINT ( 'NONE',  ( 58.81500316096885683, 85.31629705828423482, -14.27754138227609104 ) ) ;
#5565=CARTESIAN_POINT ( 'NONE',  ( 78.90361596372913766, 57.31366504278730645, -2.008240199223393141 ) ) ;
#5584=CARTESIAN_POINT ( 'NONE',  ( 57.60739473171254588, 76.56951856390271871, -18.44378120684195110 ) ) ;
#5612=CARTESIAN_POINT ( 'NONE',  ( 78.05328906524978549, 56.09831538232894843, -3.025823995327163729 ) ) ;
#5623=CARTESIAN_POINT ( 'NONE',  ( 76.76433846554481022, 54.31953569828399964, -19.93927737394622213 ) ) ;
#5652=CARTESIAN_POINT ( 'NONE',  ( 82.93675860350933249, 62.01530615766962029, -25.34918193670429076 ) ) ;
#5664=VERTEX_POINT ( 'NONE', #188 ) ;
#5688=CARTESIAN_POINT ( 'NONE',  ( 61.57468973143931379, 74.87077495648827608, -20.95977551465545119 ) ) ;
#5728=AXIS2_PLACEMENT_3D ( 'NONE', #9077, #18947, #10886 ) ;
#5808=VERTEX_POINT ( 'NONE', #18923 ) ;
#5812=B_SPLINE_CURVE_WITH_KNOTS ( 'NONE', 3,
 ( #3003, #16243, #1417, #4990, #11155, #15944, #13071, #4897, #9445, #17631, #7867, #19513, #19617, #3404, #14367, #11468, #17944, #5093, #14680, #9758, #11368, #9857, #16354, #20795, #33, #6264, #6573, #12756, #16055, #1824, #134, #7966, #8270, #17842, #3309, #3110, #12971, #19218, #11271, #17740, #14781, #235, #9558, #4689, #6675, #1719, #1518, #14468, #20891, #13172, #17526, #6366, #12862, #19316 ),
 .UNSPECIFIED., .F., .F.,
 ( 4, 2, 2, 2, 2, 2, 2, 2, 2, 2, 2, 2, 2, 2, 2, 2, 2, 2, 2, 2, 2, 2, 2, 2, 2, 2, 4 ),
 ( 0.03645627031100262538, 0.03721136074309028957, 0.03796645117517795376, 0.03872154160726561795, 0.03947663203935328213, 0.04098681290352861051, 0.04174190333561626082, 0.04249699376770391113, 0.04551735549605451236, 0.04853771722440511360, 0.05155807895275570096, 0.05457844068110630220, 0.06061916413780750468, 0.06363952586615809204, 0.06665988759450866552, 0.06968024932285923900, 0.07119043018703451187, 0.07270061105120978473, 0.07345570148329741422, 0.07421079191538507147, 0.07496588234747270096, 0.07572097277956035821, 0.07723115364373561720, 0.07874133450791087618, 0.08176169623626142191, 0.08327187710043668090, 0.08478205796461193988 ),
 .UNSPECIFIED. ) ;
#5813=AXIS2_PLACEMENT_3D ( 'NONE', #18777, #4250, #18983 ) ;
#5827=CARTESIAN_POINT ( 'NONE',  ( 82.07917159011968522, 61.14026859234759570, -0.08095729490022955666 ) ) ;
#5872=EDGE_CURVE ( 'NONE', #17011, #2714, #6067, .T. ) ;
#5882=CARTESIAN_POINT ( 'NONE',  ( 79.36047190431955300, 49.50000000000057554, -12.02697745110878280 ) ) ;
#5928=CARTESIAN_POINT ( 'NONE',  ( 81.62617710402389548, 62.35908199265414709, 0.2316258051034030541 ) ) ;
#5953=CYLINDRICAL_SURFACE ( 'NONE', #3443, 9.999999999999994671 ) ;
#5962=UNCERTAINTY_MEASURE_WITH_UNIT (LENGTH_MEASURE( 1.000000000000000082E-05 ), #19886, 'distance_accuracy_value', 'NONE');
#6023=CARTESIAN_POINT ( 'NONE',  ( 69.76445162107610543, 76.82718752816320773, -23.28021896557464387 ) ) ;
#6034=CARTESIAN_POINT ( 'NONE',  ( 79.10508859364674095, 67.76772306032525250, 0.2307413371220972953 ) ) ;
#6052=B_SPLINE_CURVE_WITH_KNOTS ( 'NONE', 3,
 ( #18369, #4042, #20060, #20156, #8710, #18259, #13497, #3725, #3943, #5522, #8816, #11691, #15317, #10075, #2359, #2047, #13706, #773, #13287, #7224, #15002, #13606, #5623, #15209, #3835, #8391, #5204, #10181, #5305, #16879, #660, #8500, #16987, #10498, #10286, #12110, #16673, #11796, #18576, #12010, #19943, #5411, #14893, #8605, #354, #460, #6801, #18157, #2155, #15102 ),
 .UNSPECIFIED., .F., .F.,
 ( 4, 2, 2, 2, 2, 2, 2, 2, 2, 2, 2, 2, 2, 2, 2, 2, 2, 2, 2, 2, 2, 2, 2, 2, 4 ),
 ( 0.1153743516471457259, 0.1159013919239667845, 0.1164284322007878569, 0.1169554724776089155, 0.1174825127544299741, 0.1185365933080721051, 0.1195906738617142223, 0.1216988349689984705, 0.1238069960762827049, 0.1259151571835669670, 0.1280233182908512013, 0.1301314793981354634, 0.1322396405054196977, 0.1332937210590618149, 0.1343478016127039598, 0.1364559627199881942, 0.1375100432736303391, 0.1385641238272724562, 0.1406722849345567183, 0.1417263654881988355, 0.1427804460418409527, 0.1448886071491252148, 0.1459426877027673319, 0.1469967682564094491, 0.1491049293636936834 ),
 .UNSPECIFIED. ) ;
#6056=ORIENTED_EDGE ( 'NONE', *, *, #10790, .F. ) ;
#6059=FACE_OUTER_BOUND ( 'NONE', #8108, .T. ) ;
#6067=B_SPLINE_CURVE_WITH_KNOTS ( 'NONE', 3,
 ( #19531, #17959, #11385, #16466, #14798, #1638, #9973, #19431, #17862, #13297, #16169, #2055, #3530, #8078, #1950, #250, #8399, #14900, #19743, #9776, #3329, #6489, #8512, #16261, #1742, #5212, #15011, #149, #3428, #8189, #14695, #13090, #6695, #11701, #50, #364, #6590, #10083, #5114, #11485, #9877, #6912, #16370, #14587, #18165, #12986, #1847, #16573, #468, #13193, #13397, #11598 ),
 .UNSPECIFIED., .F., .F.,
 ( 4, 2, 2, 2, 2, 2, 2, 2, 2, 2, 2, 2, 2, 2, 2, 2, 2, 2, 2, 2, 2, 2, 2, 2, 2, 4 ),
 ( 0.04446192691180363837, 0.04521014590794605881, 0.04595836490408848618, 0.04745480289637336868, 0.04895124088865825118, 0.05044767888094312674, 0.05344055486551287093, 0.05643343085008261512, 0.06241918281922204104, 0.06541205880379177828, 0.06840493478836148777, 0.07139781077293121114, 0.07439068675750092063, 0.07588712474978578926, 0.07738356274207063012, 0.07813178173821305750, 0.07888000073435547099, 0.08037643872664032574, 0.08112465772278276699, 0.08187287671892518048, 0.08262109571506760786, 0.08336931471121003523, 0.08486575270349486222, 0.08636219069577970309, 0.08935506668034937094, 0.09234794266491903880 ),
 .UNSPECIFIED. ) ;
#6128=CARTESIAN_POINT ( 'NONE',  ( 64.92628429094538944, 80.60227088397526529, -21.04771496906974804 ) ) ;
#6140=CARTESIAN_POINT ( 'NONE',  ( 79.29870457202490286, 66.51502123048413750, 0.4125900521836811663 ) ) ;
#6226=( NAMED_UNIT ( * ) PLANE_ANGLE_UNIT ( ) SI_UNIT ( $, .RADIAN. ) );
#6240=CARTESIAN_POINT ( 'NONE',  ( 80.96799772285972097, 65.13527580443323473, 0.5013398903319724598 ) ) ;
#6264=CARTESIAN_POINT ( 'NONE',  ( 74.48213423432167701, 73.05094370868849296, -0.3751272339344335349 ) ) ;
#6333=CARTESIAN_POINT ( 'NONE',  ( 80.91816734822852197, 65.18632510224837517, -25.49999999999999645 ) ) ;
#6340=CARTESIAN_POINT ( 'NONE',  ( 58.93693122809133911, 85.22261901257984107, -10.32461968670469865 ) ) ;
#6358=CARTESIAN_POINT ( 'NONE',  ( 58.59160831385305812, 85.48790580761031777, -13.02075998189842743 ) ) ;
#6365=CARTESIAN_POINT ( 'NONE',  ( 105.7973891242897650, 30.70991617951901276, -12.50000000000000000 ) ) ;
#6366=CARTESIAN_POINT ( 'NONE',  ( 81.36345691634956268, 55.21002353147210329, -2.349880481535979282 ) ) ;
#6397=AXIS2_PLACEMENT_3D ( 'NONE', #3565, #20304, #4093 ) ;
#6441=CARTESIAN_POINT ( 'NONE',  ( 62.46278923780241144, 78.25414160106842587, -9.766604451679548049 ) ) ;
#6489=CARTESIAN_POINT ( 'NONE',  ( 60.01640235382483013, 75.53995351896973887, -4.869773649086239331 ) ) ;
#6538=CARTESIAN_POINT ( 'NONE',  ( 80.22377123718597147, 65.83756043191739593, -25.47379904941673345 ) ) ;
#6547=CARTESIAN_POINT ( 'NONE',  ( 63.96297526125024291, 77.36452158080264496, -7.208114797878260482 ) ) ;
#6550=ADVANCED_FACE ( 'NONE', ( #9310 ), #15815, .F. ) ;
#6573=CARTESIAN_POINT ( 'NONE',  ( 75.24208973902655373, 72.42691426209449901, -0.2122651547815246897 ) ) ;
#6575=CARTESIAN_POINT ( 'NONE',  ( 76.31847140867067480, 53.71537708853300330, -19.03182057956520978 ) ) ;
#6580=ORIENTED_EDGE ( 'NONE', *, *, #2816, .T. ) ;
#6590=CARTESIAN_POINT ( 'NONE',  ( 54.32368702807821137, 77.96689879364747355, -13.45758936859397004 ) ) ;
#6611=CARTESIAN_POINT ( 'NONE',  ( 78.29269775295045974, 67.14660545764391486, -25.32607527901491196 ) ) ;
#6620=CARTESIAN_POINT ( 'NONE',  ( 115.7566812678108050, 36.45991617951907671, -12.49999999999999822 ) ) ;
#6631=LINE ( 'NONE', #13125, #15293 ) ;
#6637=CARTESIAN_POINT ( 'NONE',  ( 81.06711713768373784, 65.00000000000000000, 0.4999999999999962252 ) ) ;
#6650=CARTESIAN_POINT ( 'NONE',  ( 62.58256123368390433, 78.18905788646169697, -12.55308404828634039 ) ) ;
#6667=ADVANCED_FACE ( 'NONE', ( #9629 ), #1591, .T. ) ;
#6675=CARTESIAN_POINT ( 'NONE',  ( 82.90799867058008488, 61.47212875548994049, 0.2523705075321406865 ) ) ;
#6678=CARTESIAN_POINT ( 'NONE',  ( 79.43779261569734729, 49.71110166847581979, -14.71424312708910698 ) ) ;
#6695=CARTESIAN_POINT ( 'NONE',  ( 54.38430900759308884, 77.94115371992377561, -11.24098572673000795 ) ) ;
#6713=CARTESIAN_POINT ( 'NONE',  ( 79.89995321854216570, 66.11592257250090654, -25.45829505270997117 ) ) ;
#6754=CARTESIAN_POINT ( 'NONE',  ( 61.60468526918592858, 83.16973256007099735, -6.383283800364179861 ) ) ;
#6779=VERTEX_POINT ( 'NONE', #10428 ) ;
#6788=CARTESIAN_POINT ( 'NONE',  ( 79.70372278314360415, 50.44095208298563904, -16.99510208773339315 ) ) ;
#6793=ADVANCED_BREP_SHAPE_REPRESENTATION ( '', ( #10712, #18233 ), #16874 ) ;
#6795=ORIENTED_EDGE ( 'NONE', *, *, #12686, .T. ) ;
#6801=CARTESIAN_POINT ( 'NONE',  ( 77.00536975482934565, 54.64809360459321397, -4.630024151736636284 ) ) ;
#6828=ADVANCED_FACE ( 'NONE', ( #5336 ), #4084, .T. ) ;
#6835=CARTESIAN_POINT ( 'NONE',  ( 82.28441920437502688, 62.16931913188273739, -25.19187085580666974 ) ) ;
#6843=DIRECTION ( 'NONE',  ( 0.2588190451025150773, 0.9659258262890698665, 8.659560562354927928E-17 ) ) ;
#6851=CARTESIAN_POINT ( 'NONE',  ( 81.73379619358640014, 63.34273602762666400, 0.3959381786365755440 ) ) ;
#6869=CARTESIAN_POINT ( 'NONE',  ( 58.58021009698714465, 85.49666042193958049, -12.14404289180734686 ) ) ;
#6873=DIRECTION ( 'NONE',  ( 0.5000000000000045519, -0.8660254037844362651, 0.000000000000000000 ) ) ;
#6898=CARTESIAN_POINT ( 'NONE',  ( 77.93373660234723843, 52.03134620786124032, -13.52073087868893353 ) ) ;
#6912=CARTESIAN_POINT ( 'NONE',  ( 54.95391741498237081, 77.69916480981964924, -15.28953269010268734 ) ) ;
#6925=CARTESIAN_POINT ( 'NONE',  ( 79.81850713789391705, 50.75766720200975612, -17.68144038527332285 ) ) ;
#6931=CARTESIAN_POINT ( 'NONE',  ( 82.94363963020224162, 62.33598545253519774, -25.40129762469373631 ) ) ;
#6952=CARTESIAN_POINT ( 'NONE',  ( 80.83948132674352394, 60.42342883285770938, -0.3256906176670446573 ) ) ;
#6953=DIRECTION ( 'NONE',  ( 1.000000000000000000, -0.000000000000000000, -0.000000000000000000 ) ) ;
#6973=CARTESIAN_POINT ( 'NONE',  ( 54.27365823804359479, 77.98814336746363551, -11.88731395325653040 ) ) ;
#6997=CARTESIAN_POINT ( 'NONE',  ( 82.92574498128803384, 61.78441515947673679, 0.3082669428048712135 ) ) ;
#7029=VERTEX_POINT ( 'NONE', #444 ) ;
#7034=CARTESIAN_POINT ( 'NONE',  ( 82.74544973607177667, 63.95453548303478897, -25.58011531139869632 ) ) ;
#7041=CARTESIAN_POINT ( 'NONE',  ( 79.51181077588671542, 55.06802793803193197, -20.92898252978093865 ) ) ;
#7064=CARTESIAN_POINT ( 'NONE',  ( 104.7973891242897650, 32.44196698708787352, -12.50000000000000000 ) ) ;
#7082=CARTESIAN_POINT ( 'NONE',  ( 54.32373986521573528, 77.96687596514310314, -13.46425722430111982 ) ) ;
#7093=CIRCLE ( 'NONE', #6397, 9.999999999999994671 ) ;
#7106=CARTESIAN_POINT ( 'NONE',  ( 81.10922206268567436, 58.43639235104441809, -1.256738101660075380 ) ) ;
#7109=CARTESIAN_POINT ( 'NONE',  ( 79.45107170937350816, 54.94789128765694386, -4.214488722304810864 ) ) ;
#7121=EDGE_LOOP ( 'NONE', ( #8401, #19843, #969, #14598 ) ) ;
#7140=CARTESIAN_POINT ( 'NONE',  ( 82.32810266468291616, 65.12101312253520291, -25.63465024353788735 ) ) ;
#7146=CARTESIAN_POINT ( 'NONE',  ( 81.82243405374090628, 65.98882302804530298, -25.63369653231234224 ) ) ;
#7147=CARTESIAN_POINT ( 'NONE',  ( 59.14661261761333577, 85.06148897809092091, -15.22085364341173275 ) ) ;
#7179=DIRECTION ( 'NONE',  ( 0.5000000000000041078, -0.8660254037844361541, 0.000000000000000000 ) ) ;
#7187=CARTESIAN_POINT ( 'NONE',  ( 56.96510188438568889, 76.84332181286218599, -17.86482079344752094 ) ) ;
#7224=CARTESIAN_POINT ( 'NONE',  ( 77.94019217027455682, 55.93687283931910770, -21.83955200455485723 ) ) ;
#7246=CARTESIAN_POINT ( 'NONE',  ( 80.61604135543218774, 67.52081658169056766, -25.56477633425226159 ) ) ;
#7250=CARTESIAN_POINT ( 'NONE',  ( 49.86389338619021316, 127.5895726428436205, -12.50000000000000000 ) ) ;
#7252=CARTESIAN_POINT ( 'NONE',  ( 78.40252712997106244, 56.59081475091886659, -22.42589158092872026 ) ) ;
#7284=CARTESIAN_POINT ( 'NONE',  ( 58.68839529967456059, 85.41356074434793300, -13.73659394825620872 ) ) ;
#7313=CARTESIAN_POINT ( 'NONE',  ( 82.56388879349609056, 59.39730502837629444, -0.2907553109146409076 ) ) ;
#7325=FACE_OUTER_BOUND ( 'NONE', #4673, .T. ) ;
#7414=CARTESIAN_POINT ( 'NONE',  ( 82.68772507326825405, 59.96207871578241821, -0.1148040406626176790 ) ) ;
#7483=AXIS2_PLACEMENT_3D ( 'NONE', #18172, #15017, #13511 ) ;
#7513=DIRECTION ( 'NONE',  ( -0.7377723590286303645, 0.4392898442850237672, 0.5125586590443765855 ) ) ;
#7525=CARTESIAN_POINT ( 'NONE',  ( 82.70822966583139646, 64.11489447924186891, 0.5923196681384729212 ) ) ;
#7620=CARTESIAN_POINT ( 'NONE',  ( 61.57468973143931379, 78.66722686282992072, -24.21353532798446651 ) ) ;
#7632=CARTESIAN_POINT ( 'NONE',  ( 80.83364148849122444, 66.21898444903385439, 0.4528609240599802965 ) ) ;
#7654=DIRECTION ( 'NONE',  ( -0.8660254037844362651, -0.5000000000000042188, 0.000000000000000000 ) ) ;
#7658=DIRECTION ( 'NONE',  ( 1.000000000000000000, -0.000000000000000000, -0.000000000000000000 ) ) ;
#7666=CARTESIAN_POINT ( 'NONE',  ( 64.92628429094538944, 80.60227088397526529, -21.04771496906974448 ) ) ;
#7726=ADVANCED_FACE ( 'NONE', ( #15065 ), #4424, .T. ) ;
#7735=CARTESIAN_POINT ( 'NONE',  ( 82.29545726055718546, 62.24665149762746807, 0.2089934920557551534 ) ) ;
#7790=AXIS2_PLACEMENT_3D ( 'NONE', #9122, #10501, #14144 ) ;
#7792=DIRECTION ( 'NONE',  ( 1.000000000000000000, -0.000000000000000000, -0.000000000000000000 ) ) ;
#7832=CARTESIAN_POINT ( 'NONE',  ( 62.36299956745850892, 74.53177739387973588, -21.35531421961401222 ) ) ;
#7838=CARTESIAN_POINT ( 'NONE',  ( 82.25636457018906356, 63.72284541912095079, 0.4406977701249564228 ) ) ;
#7867=CARTESIAN_POINT ( 'NONE',  ( 59.65508358009556389, 84.67062659264655622, -8.767208989671093633 ) ) ;
#7901=DIRECTION ( 'NONE',  ( -0.5000000000000045519, 0.8660254037844360431, 0.000000000000000000 ) ) ;
#7916=EDGE_CURVE ( 'NONE', #13099, #7029, #9805, .T. ) ;
#7936=CARTESIAN_POINT ( 'NONE',  ( 81.27003798075334373, 65.71846927405951533, 0.4875263538762131255 ) ) ;
#7966=CARTESIAN_POINT ( 'NONE',  ( 80.73554840084692330, 67.38772768083256892, 0.5743335871849057916 ) ) ;
#8002=LINE ( 'NONE', #16090, #12633 ) ;
#8034=CARTESIAN_POINT ( 'NONE',  ( 62.76000446352012574, 78.08535740683855408, -12.62392526639253632 ) ) ;
#8078=CARTESIAN_POINT ( 'NONE',  ( 72.75533871425699317, 69.93577090895743709, -0.4654751680537443925 ) ) ;
#8096=CARTESIAN_POINT ( 'NONE',  ( 77.47201823384298791, 70.53308754211151665, -25.18754646355691307 ) ) ;
#8106=CARTESIAN_POINT ( 'NONE',  ( 79.36047190431935405, 49.50000000000002842, -12.49999999998710898 ) ) ;
#8108=EDGE_LOOP ( 'NONE', ( #13567, #15636, #18055, #12273 ) ) ;
#8141=CARTESIAN_POINT ( 'NONE',  ( 55.75516069692580601, 77.35848107071853974, -8.459772044266193447 ) ) ;
#8155=DIRECTION ( 'NONE',  ( 1.000000000000000000, -0.000000000000000000, -0.000000000000000000 ) ) ;
#8174=CARTESIAN_POINT ( 'NONE',  ( 78.08475988003900170, 52.31638249278350372, -9.615814618914521716 ) ) ;
#8189=CARTESIAN_POINT ( 'NONE',  ( 54.68102985684372896, 77.81511808474795089, -10.30370030985628027 ) ) ;
#8207=CARTESIAN_POINT ( 'NONE',  ( 70.65802621385911664, 70.89520902279555514, -24.10184437820831960 ) ) ;
#8213=CARTESIAN_POINT ( 'NONE',  ( 38.17255043510031953, 120.8395726428435637, -12.49999999999999822 ) ) ;
#8247=CARTESIAN_POINT ( 'NONE',  ( 66.25714559803427051, 75.99906101403284708, -4.941591886955796653 ) ) ;
#8256=AXIS2_PLACEMENT_3D ( 'NONE', #7620, #7513, #955 ) ;
#8270=CARTESIAN_POINT ( 'NONE',  ( 81.06335414937042572, 67.01023635845230331, 0.5981178230952700625 ) ) ;
#8273=CARTESIAN_POINT ( 'NONE',  ( 75.61984849132328179, 52.78225778306437377, -16.94885618148015993 ) ) ;
#8298=VERTEX_POINT ( 'NONE', #19138 ) ;
#8355=CARTESIAN_POINT ( 'NONE',  ( 69.95688439207881970, 76.67563175530182207, -1.651812347404341796 ) ) ;
#8383=CARTESIAN_POINT ( 'NONE',  ( 76.24641241968245708, 53.61856141616145521, -6.137685929381720307 ) ) ;
#8391=CARTESIAN_POINT ( 'NONE',  ( 75.73459986189040194, 52.93517924382847895, -17.35279103460518968 ) ) ;
#8399=CARTESIAN_POINT ( 'NONE',  ( 67.54734661231900361, 72.27942328892467572, -1.687414245825497261 ) ) ;
#8401=ORIENTED_EDGE ( 'NONE', *, *, #7916, .F. ) ;
#8411=CARTESIAN_POINT ( 'NONE',  ( 81.83695616705894338, 65.97962712285851694, -25.63559049685116165 ) ) ;
#8416=CARTESIAN_POINT ( 'NONE',  ( 77.64566045588958332, 55.52805080504859347, -21.41780359453167293 ) ) ;
#8455=CARTESIAN_POINT ( 'NONE',  ( 62.45904372457708575, 78.26118437974417930, -12.42744951105453488 ) ) ;
#8491=CARTESIAN_POINT ( 'NONE',  ( 75.38193994203784598, 52.46588049713438551, -15.95886351416976900 ) ) ;
#8500=CARTESIAN_POINT ( 'NONE',  ( 75.05058039824011473, 52.02675804008249827, -13.40131898612561301 ) ) ;
#8512=CARTESIAN_POINT ( 'NONE',  ( 59.22717251798539451, 75.87775315904988815, -5.353841392320322079 ) ) ;
#8533=CARTESIAN_POINT ( 'NONE',  ( 82.11984465641647546, 64.23705030780924119, -25.48156911047034612 ) ) ;
#8572=CARTESIAN_POINT ( 'NONE',  ( 62.17916131348992081, 78.42313103979506650, -13.88866078518543112 ) ) ;
#8598=CARTESIAN_POINT ( 'NONE',  ( 75.23666811385876940, 52.27308886237457841, -15.20134910407188400 ) ) ;
#8605=CARTESIAN_POINT ( 'NONE',  ( 76.47376643088200865, 53.92683595214138137, -5.681768602789493805 ) ) ;
#8630=CARTESIAN_POINT ( 'NONE',  ( 81.85908840240438167, 56.78121513735760573, -23.59847208966338528 ) ) ;
#8636=CARTESIAN_POINT ( 'NONE',  ( 81.59473887788738011, 64.10409879185415605, -25.47155011481813602 ) ) ;
#8677=CARTESIAN_POINT ( 'NONE',  ( 54.37566476943453608, 77.94482555308654526, -13.72387178829551502 ) ) ;
#8699=CARTESIAN_POINT ( 'NONE',  ( 81.85522543128666939, 56.76562253233274902, -1.406549998271479751 ) ) ;
#8710=CARTESIAN_POINT ( 'NONE',  ( 81.52759066145694078, 64.25397585761884045, -25.47962019146266499 ) ) ;
#8735=CARTESIAN_POINT ( 'NONE',  ( 80.72516319149150377, 53.31353001781401701, -21.13911636830589558 ) ) ;
#8740=CARTESIAN_POINT ( 'NONE',  ( 82.12886169804700387, 61.33916772676509055, -24.97880947958990561 ) ) ;
#8742=CARTESIAN_POINT ( 'NONE',  ( 60.52928988819383704, 83.99806976322641106, -17.46522718495289439 ) ) ;
#8781=CARTESIAN_POINT ( 'NONE',  ( 62.17277006171050147, 78.42718308225904877, -13.70364326203602268 ) ) ;
#8782=EDGE_CURVE ( 'NONE', #6779, #20850, #5812, .T. ) ;
#8816=CARTESIAN_POINT ( 'NONE',  ( 81.63447678882555181, 62.38330499993598011, -25.23821314459116394 ) ) ;
#8841=CARTESIAN_POINT ( 'NONE',  ( 79.36047190431935405, 49.50000000000002842, -12.49999999998710898 ) ) ;
#8846=CARTESIAN_POINT ( 'NONE',  ( 82.73391158952136948, 64.01818219908709295, -25.58603017124621815 ) ) ;
#8847=CARTESIAN_POINT ( 'NONE',  ( 58.88613401674517434, 85.26164830632635017, -14.51790671232051899 ) ) ;
#8885=CARTESIAN_POINT ( 'NONE',  ( 59.47741263991522942, 75.77081037196482782, -19.82212451566851286 ) ) ;
#8912=CARTESIAN_POINT ( 'NONE',  ( 80.71088083322737816, 60.18095083263530398, -0.4163648238935768187 ) ) ;
#8963=CARTESIAN_POINT ( 'NONE',  ( 81.68654525303921332, 62.66781674343961583, 0.2910019319276673788 ) ) ;
#8968=EDGE_CURVE ( 'NONE', #3901, #19292, #20675, .T. ) ;
#8982=CARTESIAN_POINT ( 'NONE',  ( 64.57205371728791476, 77.00255147951500589, -18.47244162738281048 ) ) ;
#9012=CARTESIAN_POINT ( 'NONE',  ( 80.14546250568827190, 56.34553042421615743, -2.766056647043495076 ) ) ;
#9068=CARTESIAN_POINT ( 'NONE',  ( 79.53442306383087157, 49.97558790125707873, -9.251858224647309115 ) ) ;
#9077=CARTESIAN_POINT ( 'NONE',  ( 86.00000000000000000, 65.00000000000000000, -12.50000000000000000 ) ) ;
#9093=AXIS2_PLACEMENT_3D ( 'NONE', #1503, #9543, #9846 ) ;
#9108=CARTESIAN_POINT ( 'NONE',  ( 82.94070292489149665, 62.10228613400511932, 0.3639711883102479395 ) ) ;
#9122=CARTESIAN_POINT ( 'NONE',  ( 105.7973891242897650, 30.70991617951901986, -12.50000000000000000 ) ) ;
#9165=VECTOR ( 'NONE', #6953, 1000.000000000000000 ) ;
#9215=CARTESIAN_POINT ( 'NONE',  ( 81.82126993650646796, 64.90558118418934441, 0.5045236030688061701 ) ) ;
#9242=ORIENTED_EDGE ( 'NONE', *, *, #490, .F. ) ;
#9285=ORIENTED_EDGE ( 'NONE', *, *, #15499, .T. ) ;
#9310=FACE_OUTER_BOUND ( 'NONE', #20443, .T. ) ;
#9313=CARTESIAN_POINT ( 'NONE',  ( 81.31380233296179938, 64.67425244115396765, 0.4979624178218136077 ) ) ;
#9330=CARTESIAN_POINT ( 'NONE',  ( 62.09798184194390558, 82.78955810596320930, -19.07905325425590704 ) ) ;
#9407=( LENGTH_UNIT ( ) NAMED_UNIT ( * ) SI_UNIT ( .MILLI., .METRE. ) );
#9422=CARTESIAN_POINT ( 'NONE',  ( 67.37294370578848657, 72.35496154219596576, -1.763419216299827008 ) ) ;
#9445=CARTESIAN_POINT ( 'NONE',  ( 59.12602517596783969, 85.07731064195019144, -9.828416369996476831 ) ) ;
#9527=CARTESIAN_POINT ( 'NONE',  ( 82.79352064649921772, 63.77227335278520570, 0.5678441448316937645 ) ) ;
#9543=DIRECTION ( 'NONE',  ( 1.000000000000000000, -0.000000000000000000, -0.000000000000000000 ) ) ;
#9556=EDGE_LOOP ( 'NONE', ( #4428, #16176, #13374, #17947, #9242, #14046 ) ) ;
#9558=CARTESIAN_POINT ( 'NONE',  ( 82.92989559899719154, 62.71207119171138800, 0.4539515997919767454 ) ) ;
#9590=B_SPLINE_CURVE_WITH_KNOTS ( 'NONE', 3,
 ( #2625, #17241, #2832, #10557, #1027, #20617, #18836, #19049, #9068, #18733, #20414, #10986, #5882, #12377 ),
 .UNSPECIFIED., .F., .F.,
 ( 4, 2, 2, 2, 2, 2, 4 ),
 ( 0.08478205796461193988, 0.08763025155739845307, 0.09047844515018496625, 0.09190254194657822284, 0.09332663874297149331, 0.09475073553936474990, 0.09617483233575800650 ),
 .UNSPECIFIED. ) ;
#9629=FACE_OUTER_BOUND ( 'NONE', #2724, .T. ) ;
#9632=CARTESIAN_POINT ( 'NONE',  ( 54.35552982649267051, 77.95337578947557233, -11.36981949127928893 ) ) ;
#9633=EDGE_CURVE ( 'NONE', #13156, #5664, #13602, .T. ) ;
#9725=CARTESIAN_POINT ( 'NONE',  ( 81.06711713768373784, 65.00000000000000000, -25.50000000000000000 ) ) ;
#9735=CARTESIAN_POINT ( 'NONE',  ( 62.29739936921044574, 78.35542098874827843, -12.12431711150143521 ) ) ;
#9758=CARTESIAN_POINT ( 'NONE',  ( 65.44812640818317107, 80.19785434853127981, -3.638783230584851758 ) ) ;
#9761=CARTESIAN_POINT ( 'NONE',  ( 77.92638923178418509, 52.01750209009090042, -11.67654819968911717 ) ) ;
#9776=CARTESIAN_POINT ( 'NONE',  ( 62.45290926645331098, 74.49313803559309122, -3.604012042188190268 ) ) ;
#9796=CARTESIAN_POINT ( 'NONE',  ( 66.81417725909253136, 79.13633915520293272, -22.06525532588372585 ) ) ;
#9805=LINE ( 'NONE', #6620, #332 ) ;
#9815=AXIS2_PLACEMENT_3D ( 'NONE', #2266, #17208, #20169 ) ;
#9833=CARTESIAN_POINT ( 'NONE',  ( 63.34582467611540579, 77.73072509497566784, -8.044670883999552657 ) ) ;
#9846=DIRECTION ( 'NONE',  ( 0.000000000000000000, 0.000000000000000000, -1.000000000000000000 ) ) ;
#9857=CARTESIAN_POINT ( 'NONE',  ( 67.66310225583265492, 78.47357137787466286, -2.555409790234332235 ) ) ;
#9861=CARTESIAN_POINT ( 'NONE',  ( 75.90040729020685717, 53.15606728486817190, -7.041156951942071807 ) ) ;
#9877=CARTESIAN_POINT ( 'NONE',  ( 54.74529948059490891, 77.78781281343189846, -14.84991977410729191 ) ) ;
#9885=ADVANCED_FACE ( 'NONE', ( #6059 ), #5953, .T. ) ;
#9896=CARTESIAN_POINT ( 'NONE',  ( 61.57468973143931379, 74.87077495648827608, -20.95977551465545119 ) ) ;
#9936=CARTESIAN_POINT ( 'NONE',  ( 64.60297720430702384, 80.85304810415020427, -4.137593906014268796 ) ) ;
#9957=CARTESIAN_POINT ( 'NONE',  ( 75.38983945845171775, 52.47636342738726256, -9.003451077243985523 ) ) ;
#9973=CARTESIAN_POINT ( 'NONE',  ( 79.20327082793765783, 66.58182770179300292, 0.4060056306182541763 ) ) ;
#9988=CARTESIAN_POINT ( 'NONE',  ( 82.53324728627625007, 64.66165602865051198, -25.62270589083005845 ) ) ;
#9991=CARTESIAN_POINT ( 'NONE',  ( 80.95562266652501648, 67.15461460196840449, -25.59299666572612963 ) ) ;
#10019=EDGE_CURVE ( 'NONE', #5664, #7029, #10265, .T. ) ;
#10037=CARTESIAN_POINT ( 'NONE',  ( 58.19665357825395802, 76.31805631966230408, -6.092558036382285991 ) ) ;
#10052=DIRECTION ( 'NONE',  ( 0.5000000000000045519, -0.8660254037844362651, 0.000000000000000000 ) ) ;
#10067=CARTESIAN_POINT ( 'NONE',  ( 80.60295752769052058, 52.96396996839209237, -20.75661811798801892 ) ) ;
#10075=CARTESIAN_POINT ( 'NONE',  ( 80.90185716406490712, 60.51308707325554792, -24.71776202822431046 ) ) ;
#10083=CARTESIAN_POINT ( 'NONE',  ( 54.42754686098177075, 77.92279056475767618, -13.93489572546247857 ) ) ;
#10096=CARTESIAN_POINT ( 'NONE',  ( 81.55002576568772099, 66.38583373074199301, -25.62495068049236835 ) ) ;
#10102=CARTESIAN_POINT ( 'NONE',  ( 78.66618490269718222, 56.96778211784575774, -22.73333863286613266 ) ) ;
#10123=CARTESIAN_POINT ( 'NONE',  ( 78.05328906524978549, 52.67459052937854835, 0.6180898526239277935 ) ) ;
#10140=CARTESIAN_POINT ( 'NONE',  ( 62.90137823179582455, 78.00269638309853804, -12.54667390848797837 ) ) ;
#10171=CARTESIAN_POINT ( 'NONE',  ( 78.40297945836096005, 52.91941870341079834, -7.572629818528286094 ) ) ;
#10181=CARTESIAN_POINT ( 'NONE',  ( 75.48021121295072078, 52.59641686382532555, -16.40691147115069626 ) ) ;
#10212=CARTESIAN_POINT ( 'NONE',  ( 80.02304891312839175, 59.01526275525436915, -24.05071924315015153 ) ) ;
#10229=CARTESIAN_POINT ( 'NONE',  ( 81.54035229546286700, 64.23212122210442487, 0.4788660375907791700 ) ) ;
#10231=CARTESIAN_POINT ( 'NONE',  ( 86.00000000000000000, 65.00000000000000000, -2.500000000000005773 ) ) ;
#10249=CARTESIAN_POINT ( 'NONE',  ( 54.25673667531765432, 77.99532872960556062, -12.93714471232228647 ) ) ;
#10257=CARTESIAN_POINT ( 'NONE',  ( 86.00000000000000000, 65.00000000000000000, 0.4999999999999970024 ) ) ;
#10265=LINE ( 'NONE', #12197, #10887 ) ;
#10286=CARTESIAN_POINT ( 'NONE',  ( 75.03375843245487431, 52.00451211173042054, -12.01334687468304985 ) ) ;
#10308=CARTESIAN_POINT ( 'NONE',  ( 79.40833726504349954, 49.63029741583935106, -14.45290996621378277 ) ) ;
#10312=FACE_OUTER_BOUND ( 'NONE', #16099, .T. ) ;
#10316=CARTESIAN_POINT ( 'NONE',  ( 82.34777263834683936, 58.50307748515720618, -24.38835257526326927 ) ) ;
#10340=DIRECTION ( 'NONE',  ( 0.8660254037844358210, 0.5000000000000046629, 0.000000000000000000 ) ) ;
#10346=ADVANCED_FACE ( 'NONE', ( #20115 ), #3790, .T. ) ;
#10355=CARTESIAN_POINT ( 'NONE',  ( 62.68497280389577497, 78.12921337523277998, -12.39230198697897833 ) ) ;
#10356=ORIENTED_EDGE ( 'NONE', *, *, #2573, .F. ) ;
#10380=CARTESIAN_POINT ( 'NONE',  ( 82.87092262195501746, 61.16184052528804926, 0.1830206181285179701 ) ) ;
#10402=PRODUCT ( '60-Degree Angle Clamping Handle', '60-Degree Angle Clamping Handle', '', ( #14448 ) ) ;
#10417=CARTESIAN_POINT ( 'NONE',  ( 79.36047190431891352, 49.49999999999888445, -13.48535184266127551 ) ) ;
#10425=CARTESIAN_POINT ( 'NONE',  ( 81.66740910649770058, 62.54383302279143919, -25.26856822461360608 ) ) ;
#10428=CARTESIAN_POINT ( 'NONE',  ( 58.57586221349259858, 85.50000000000002842, -12.50000000002017231 ) ) ;
#10449=CARTESIAN_POINT ( 'NONE',  ( 78.05328906524978549, 56.09831538232894843, -3.025823995327162841 ) ) ;
#10459=CARTESIAN_POINT ( 'NONE',  ( 61.48790260083684700, 83.25974565949677242, -18.50556687427830127 ) ) ;
#10472=CARTESIAN_POINT ( 'NONE',  ( 81.10655718899290889, 54.43739570252013493, -2.927339837283823520 ) ) ;
#10486=CARTESIAN_POINT ( 'NONE',  ( 79.38331026022220271, 58.02222229763877692, -1.520680142459543305 ) ) ;
#10489=CARTESIAN_POINT ( 'NONE',  ( 77.79949723222266300, 55.74148623974197392, -3.361091198315218520 ) ) ;
#10498=CARTESIAN_POINT ( 'NONE',  ( 75.02738531498535224, 51.99608617524740595, -12.36235906538899521 ) ) ;
#10501=DIRECTION ( 'NONE',  ( 0.5000000000000045519, -0.8660254037844362651, 0.000000000000000000 ) ) ;
#10535=CARTESIAN_POINT ( 'NONE',  ( 82.63287099403851244, 64.35888726086905365, -25.60638951267676688 ) ) ;
#10553=B_SPLINE_CURVE_WITH_KNOTS ( 'NONE', 3,
 ( #19973, #2389, #12541, #9330, #5439, #8742, #15239, #15829, #692, #7147, #13636, #8847, #5550, #15346, #17933, #6358, #225, #3395 ),
 .UNSPECIFIED., .F., .F.,
 ( 4, 2, 2, 2, 2, 2, 2, 2, 4 ),
 ( 0.02406572584676644130, 0.02716336196282548646, 0.03026099807888454549, 0.03180981613691406806, 0.03335863419494358717, 0.03413304322395834672, 0.03490745225297310628, 0.03568186128198786583, 0.03645627031100262538 ),
 .UNSPECIFIED. ) ;
#10557=CARTESIAN_POINT ( 'NONE',  ( 80.21122190583011502, 51.84991952600655196, -5.522095467871776187 ) ) ;
#10576=CARTESIAN_POINT ( 'NONE',  ( 62.19646603496936166, 78.41412544775637627, -13.18179411983555660 ) ) ;
#10590=ADVANCED_FACE ( 'NONE', ( #17464 ), #2111, .T. ) ;
#10602=CARTESIAN_POINT ( 'NONE',  ( 79.96260520138829975, 55.97221593644851367, -3.110880007782513168 ) ) ;
#10603=VERTEX_POINT ( 'NONE', #1456 ) ;
#10633=AXIS2_PLACEMENT_3D ( 'NONE', #7250, #20187, #687 ) ;
#10639=EDGE_CURVE ( 'NONE', #14308, #14580, #8002, .T. ) ;
#10702=AXIS2_PLACEMENT_3D ( 'NONE', #7064, #13547, #5460 ) ;
#10705=CARTESIAN_POINT ( 'NONE',  ( 80.60135456229210149, 66.45530591845690083, 0.4295846759676194559 ) ) ;
#10711=CARTESIAN_POINT ( 'NONE',  ( 78.05328906524978549, 56.09831538232894843, -3.025823995327163729 ) ) ;
#10712=MANIFOLD_SOLID_BREP ( 'Chamfer1', #15451 ) ;
#10752=CARTESIAN_POINT ( 'NONE',  ( 93.10604617319987142, 25.69196698708779536, -12.49999999999999822 ) ) ;
#10790=EDGE_CURVE ( 'NONE', #19064, #17011, #17486, .T. ) ;
#10808=CARTESIAN_POINT ( 'NONE',  ( 81.33834232799965491, 66.66102642021321856, 0.6137031208531950055 ) ) ;
#10850=ORIENTED_EDGE ( 'NONE', *, *, #20916, .F. ) ;
#10876=LINE ( 'NONE', #20516, #14849 ) ;
#10880=AXIS2_PLACEMENT_3D ( 'NONE', #18177, #1961, #2069 ) ;
#10886=DIRECTION ( 'NONE',  ( 0.000000000000000000, 0.000000000000000000, -1.000000000000000000 ) ) ;
#10887=VECTOR ( 'NONE', #18347, 1000.000000000000114 ) ;
#10915=CARTESIAN_POINT ( 'NONE',  ( 77.98781333307499608, 70.07958826284888687, -25.26506956498398893 ) ) ;
#10926=CARTESIAN_POINT ( 'NONE',  ( 80.30982465549199389, 65.77076383589957231, 0.4787884790452578976 ) ) ;
#10986=CARTESIAN_POINT ( 'NONE',  ( 79.37186041290443939, 49.53105059404756361, -11.54859855717600325 ) ) ;
#10998=CARTESIAN_POINT ( 'NONE',  ( 115.7566812678108050, 36.45991617951909092, -12.49999999999999822 ) ) ;
#11004=ORIENTED_EDGE ( 'NONE', *, *, #18599, .T. ) ;
#11017=SHAPE_REPRESENTATION_RELATIONSHIP ( 'NONE' , 'NONE' ,  #16277, #6793 ) ;
#11022=CARTESIAN_POINT ( 'NONE',  ( 63.75189850252981216, 73.93268399900620125, -21.96684734925903726 ) ) ;
#11031=CARTESIAN_POINT ( 'NONE',  ( 77.50103995547023317, 68.94704969384721949, -0.06791703117014312452 ) ) ;
#11073=ORIENTED_EDGE ( 'NONE', *, *, #18599, .F. ) ;
#11102=EDGE_LOOP ( 'NONE', ( #6056, #12600, #20941, #3881, #4223, #19754 ) ) ;
#11132=CARTESIAN_POINT ( 'NONE',  ( 82.93030480524085135, 62.75708420226636264, 0.4611002339714860843 ) ) ;
#11155=CARTESIAN_POINT ( 'NONE',  ( 58.69187849547078883, 85.41088488089633302, -11.24813091999954295 ) ) ;
#11238=CARTESIAN_POINT ( 'NONE',  ( 69.72421256244413712, 71.31772771003116418, -23.89306908104443394 ) ) ;
#11246=CARTESIAN_POINT ( 'NONE',  ( 58.72203124118109940, 85.38772223162817454, -11.09829540933401582 ) ) ;
#11261=EDGE_LOOP ( 'NONE', ( #5504, #20615, #1137, #10850 ) ) ;
#11271=CARTESIAN_POINT ( 'NONE',  ( 82.67991938068482227, 64.19136817925864591, 0.5957706602028168819 ) ) ;
#11340=CARTESIAN_POINT ( 'NONE',  ( 62.17486404044439752, 78.42547049926599811, -11.00043863000396094 ) ) ;
#11368=CARTESIAN_POINT ( 'NONE',  ( 66.17935976187501979, 79.62987128376072121, -3.255002524965970423 ) ) ;
#11370=CARTESIAN_POINT ( 'NONE',  ( 78.20613919103151090, 52.54607637467318426, -16.26456764023157930 ) ) ;
#11385=CARTESIAN_POINT ( 'NONE',  ( 80.73926736692914119, 65.37378763963897654, 0.4957099094033766140 ) ) ;
#11404=CARTESIAN_POINT ( 'NONE',  ( 66.00360725464794598, 72.95415083537486112, -22.80269511576363328 ) ) ;
#11436=CARTESIAN_POINT ( 'NONE',  ( 64.77682424794421934, 73.48778032978390229, -22.35823834978864610 ) ) ;
#11442=CARTESIAN_POINT ( 'NONE',  ( 55.00515713082256042, 77.67739022016017714, -9.611626274830124217 ) ) ;
#11468=CARTESIAN_POINT ( 'NONE',  ( 61.33030688981697409, 83.38129477918221255, -6.619636938701232154 ) ) ;
#11470=CARTESIAN_POINT ( 'NONE',  ( 79.05205211475293936, 54.16676007582333341, -19.73373562583472562 ) ) ;
#11485=CARTESIAN_POINT ( 'NONE',  ( 54.65284698049440237, 77.82709027839986504, -14.62584647385420311 ) ) ;
#11504=( BOUNDED_SURFACE ( )  B_SPLINE_SURFACE ( 3, 2, ( 
 ( #5612, #15093, #16763 ),
 ( #2246, #10602, #863 ),
 ( #18567, #9012, #17087 ),
 ( #18672, #967, #4033 ),
 ( #10486, #13485, #8699 ),
 ( #651, #7106, #4149 ),
 ( #18458, #20355, #19932 ),
 ( #8912, #15408, #7313 ),
 ( #5400, #13594, #7414 ),
 ( #765, #5827, #549 ),
 ( #18248, #3933, #10380 ),
 ( #16663, #2144, #6997 ),
 ( #5928, #7735, #9108 ),
 ( #4663, #18883, #11132 ),
 ( #3080, #12631, #17607 ),
 ( #14338, #7838, #9527 ),
 ( #17186, #19093, #7525 ),
 ( #16029, #12430, #1490 ),
 ( #9313, #9215, #20770 ),
 ( #6240, #2774, #19192 ),
 ( #14018, #7936, #4356 ),
 ( #10926, #7632, #10808 ),
 ( #15818, #10705, #12728 ),
 ( #15609, #20460, #14234 ),
 ( #6140, #14130, #17288 ),
 ( #14439, #6034, #12525 ),
 ( #17397, #4565, #20867 ),
 ( #20665, #11031, #17503 ),
 ( #12324, #1182, #1387 ),
 ( #18779, #1077, #4253 ),
 ( #2668, #15719, #20563 ),
 ( #18986, #4464, #2876 ),
 ( #15918, #2979, #1289 ),
 ( #9422, #14858, #8355 ),
 ( #12836, #17714, #16329 ),
 ( #14655, #8247, #11657 ),
 ( #5068, #17919, #12943 ),
 ( #19395, #19696, #9936 ),
 ( #114, #6547, #13046 ),
 ( #11545, #9833, #3181 ),
 ( #14544, #7, #1908 ),
 ( #10037, #16126, #3377 ),
 ( #308, #6441, #6754 ),
 ( #13252, #5169, #1595 ),
 ( #4871, #11340, #18120 ),
 ( #16218, #19485, #3279 ),
 ( #8141, #1804, #3589 ),
 ( #3491, #17808, #16528 ),
 ( #1694, #9735, #4967 ),
 ( #11442, #14755, #2008 ),
 ( #207, #8455, #14959 ),
 ( #13145, #6650, #6340 ),
 ( #16428, #18019, #19293 ),
 ( #4764, #8034, #11246 ),
 ( #9632, #19587, #5273 ),
 ( #6973, #13565, #5482 ),
 ( #12178, #10140, #6869 ),
 ( #18222, #3685, #2219 ),
 ( #10249, #5374, #11976 ),
 ( #7082, #11763, #18433 ),
 ( #8677, #11866, #7284 ),
 ( #16634, #10355, #3902 ),
 ( #13355, #19800, #2431 ),
 ( #526, #18644, #19909 ),
 ( #16843, #4121, #15176 ),
 ( #18331, #3798, #15071 ),
 ( #628, #10576, #2326 ),
 ( #13460, #8781, #2120 ),
 ( #17062, #8572, #16740 ),
 ( #20021, #15279, #735 ),
 ( #7187, #13672, #20122 ),
 ( #5584, #12076, #10459 ),
 ( #18543, #4010, #16946 ),
 ( #8885, #15386, #838 ),
 ( #13774, #20222, #2538 ),
 ( #5688, #8982, #424 ) ),
 .UNSPECIFIED., .F., .F., .T. ) 
 B_SPLINE_SURFACE_WITH_KNOTS ( ( 4, 2, 2, 2, 2, 2, 2, 2, 2, 2, 2, 2, 2, 2, 2, 2, 2, 2, 2, 2, 2, 2, 2, 2, 2, 2, 2, 2, 2, 2, 2, 2, 2, 2, 2, 2, 2, 4 ),
 ( 3, 3 ),
 ( 0.06885390149614811772, 0.07100558591790274987, 0.07315727033965738202, 0.07530895476141200029, 0.07746063918316663244, 0.07853648139404395545, 0.07961232360492126459, 0.08068816581579857372, 0.08176400802667588286, 0.08283985023755319199, 0.08391569244843051500, 0.08499153465930783802, 0.08606737687018514715, 0.08821906129193977930, 0.09037074571369441145, 0.09467411455720366187, 0.09897748340071291229, 0.1032808522442221766, 0.1075842210877314409, 0.1097359055094860592, 0.1118875899312406913, 0.1140392743529953234, 0.1161909587747499417, 0.1172668009856272509, 0.1183426431965045739, 0.1194184854073818969, 0.1204943276182592060, 0.1215701698291365151, 0.1226460120400138243, 0.1237218542508911334, 0.1247976964617684564, 0.1258735386726457794, 0.1269493808835230886, 0.1291010653052777069, 0.1301769075161550160, 0.1312527497270323251, 0.1334044341487869711, 0.1377078029922962354 ),
 ( 0.000000000000000000, 1.000000000000000000 ),
 .UNSPECIFIED. ) 
 GEOMETRIC_REPRESENTATION_ITEM ( )  RATIONAL_B_SPLINE_SURFACE ( (
 ( 1.000000000000000000, 0.9375990638454466675, 1.000000000000000000),
 ( 1.000000000000000000, 0.9424674560013240887, 1.000000000000000000),
 ( 1.000000000000000000, 0.9472454495395411511, 1.000000000000000000),
 ( 1.000000000000000000, 0.9564605845185850663, 1.000000000000000000),
 ( 1.000000000000000000, 0.9608454732134027454, 1.000000000000000000),
 ( 1.000000000000000000, 0.9689919522595137336, 1.000000000000000000),
 ( 1.000000000000000000, 0.9727657420268004396, 1.000000000000000000),
 ( 1.000000000000000000, 0.9796074070863388661, 1.000000000000000000),
 ( 1.000000000000000000, 0.9826776977508318023, 1.000000000000000000),
 ( 1.000000000000000000, 0.9866441197506812255, 1.000000000000000000),
 ( 1.000000000000000000, 0.9878563112346668840, 1.000000000000000000),
 ( 1.000000000000000000, 0.9900012503172416212, 1.000000000000000000),
 ( 1.000000000000000000, 0.9909393653429625637, 1.000000000000000000),
 ( 1.000000000000000000, 0.9925019860915718084, 1.000000000000000000),
 ( 1.000000000000000000, 0.9931248883185653797, 1.000000000000000000),
 ( 1.000000000000000000, 0.9939517895330679531, 1.000000000000000000),
 ( 1.000000000000000000, 0.9941631134692228144, 1.000000000000000000),
 ( 1.000000000000000000, 0.9941219286420546197, 1.000000000000000000),
 ( 1.000000000000000000, 0.9938724371314660022, 1.000000000000000000),
 ( 1.000000000000000000, 0.9929677657768187782, 1.000000000000000000),
 ( 1.000000000000000000, 0.9923039779988552800, 1.000000000000000000),
 ( 1.000000000000000000, 0.9906518461315473312, 1.000000000000000000),
 ( 1.000000000000000000, 0.9896671415157215490, 1.000000000000000000),
 ( 1.000000000000000000, 0.9874184541695402162, 1.000000000000000000),
 ( 1.000000000000000000, 0.9861538891527321660, 1.000000000000000000),
 ( 1.000000000000000000, 0.9819645303139994397, 1.000000000000000000),
 ( 1.000000000000000000, 0.9786329312631978361, 1.000000000000000000),
 ( 1.000000000000000000, 0.9710304362473276552, 1.000000000000000000),
 ( 1.000000000000000000, 0.9667585549851247517, 1.000000000000000000),
 ( 1.000000000000000000, 0.9525417557630343479, 1.000000000000000000),
 ( 1.000000000000000000, 0.9412001842544890362, 1.000000000000000000),
 ( 1.000000000000000000, 0.9146347518846402735, 1.000000000000000000),
 ( 1.000000000000000000, 0.8994101094843396371, 1.000000000000000000),
 ( 1.000000000000000000, 0.8647450005962233899, 1.000000000000000000),
 ( 1.000000000000000000, 0.8453054357499633076, 1.000000000000000000),
 ( 1.000000000000000000, 0.8016942677996606870, 1.000000000000000000),
 ( 1.000000000000000000, 0.7777397233075318272, 1.000000000000000000),
 ( 1.000000000000000000, 0.7387134092132859875, 1.000000000000000000),
 ( 1.000000000000000000, 0.7251826916704574577, 1.000000000000000000),
 ( 1.000000000000000000, 0.6971304047192319331, 1.000000000000000000),
 ( 1.000000000000000000, 0.6826980669419527858, 1.000000000000000000),
 ( 1.000000000000000000, 0.6534760639743609767, 1.000000000000000000),
 ( 1.000000000000000000, 0.6386527339599178399, 1.000000000000000000),
 ( 1.000000000000000000, 0.6090832796716727504, 1.000000000000000000),
 ( 1.000000000000000000, 0.5943263318904800085, 1.000000000000000000),
 ( 1.000000000000000000, 0.5729533508074381443, 1.000000000000000000),
 ( 1.000000000000000000, 0.5659665513975454809, 1.000000000000000000),
 ( 1.000000000000000000, 0.5526995341054916633, 1.000000000000000000),
 ( 1.000000000000000000, 0.5463867916638659450, 1.000000000000000000),
 ( 1.000000000000000000, 0.5346239116712828698, 1.000000000000000000),
 ( 1.000000000000000000, 0.5291736392160848457, 1.000000000000000000),
 ( 1.000000000000000000, 0.5194015973764528615, 1.000000000000000000),
 ( 1.000000000000000000, 0.5150650454058257610, 1.000000000000000000),
 ( 1.000000000000000000, 0.5079781513294042705, 1.000000000000000000),
 ( 1.000000000000000000, 0.5052035616582067901, 1.000000000000000000),
 ( 1.000000000000000000, 0.5013339263629003062, 1.000000000000000000),
 ( 1.000000000000000000, 0.5002393203327387683, 1.000000000000000000),
 ( 1.000000000000000000, 0.4998309580985344502, 1.000000000000000000),
 ( 1.000000000000000000, 0.5005275148352900105, 1.000000000000000000),
 ( 1.000000000000000000, 0.5037041118084196745, 1.000000000000000000),
 ( 1.000000000000000000, 0.5061579591350763296, 1.000000000000000000),
 ( 1.000000000000000000, 0.5125803135669114718, 1.000000000000000000),
 ( 1.000000000000000000, 0.5165482939438740262, 1.000000000000000000),
 ( 1.000000000000000000, 0.5257728359944916496, 1.000000000000000000),
 ( 1.000000000000000000, 0.5310610287513783945, 1.000000000000000000),
 ( 1.000000000000000000, 0.5482655009316232952, 1.000000000000000000),
 ( 1.000000000000000000, 0.5614273505701570244, 1.000000000000000000),
 ( 1.000000000000000000, 0.5823794962627073524, 1.000000000000000000),
 ( 1.000000000000000000, 0.5895723009191430330, 1.000000000000000000),
 ( 1.000000000000000000, 0.6042245744574831212, 1.000000000000000000),
 ( 1.000000000000000000, 0.6117101498696801976, 1.000000000000000000),
 ( 1.000000000000000000, 0.6341532752532395012, 1.000000000000000000),
 ( 1.000000000000000000, 0.6490967219973816649, 1.000000000000000000),
 ( 1.000000000000000000, 0.6931167578513042216, 1.000000000000000000),
 ( 1.000000000000000000, 0.7213744951071011657, 1.000000000000000000),
 ( 1.000000000000000000, 0.7477234448260038358, 1.000000000000000000) ) ) 
 REPRESENTATION_ITEM ( '' )  SURFACE ( )  );
#11505=CARTESIAN_POINT ( 'NONE',  ( 72.81261327087452173, 74.40654852583290335, -24.22244567122760728 ) ) ;
#11545=CARTESIAN_POINT ( 'NONE',  ( 59.64661162979547271, 75.69814633436611473, -5.104845358893310703 ) ) ;
#11548=VERTEX_POINT ( 'NONE', #187 ) ;
#11562=DIRECTION ( 'NONE',  ( 0.8660254037844360431, 0.5000000000000044409, 0.000000000000000000 ) ) ;
#11578=CARTESIAN_POINT ( 'NONE',  ( 77.97393021361884280, 52.10713123856947249, -10.75681189255892534 ) ) ;
#11582=PRODUCT_DEFINITION ( 'UNKNOWN', '', #18932, #17218 ) ;
#11598=CARTESIAN_POINT ( 'NONE',  ( 61.57468973143931379, 74.87077495648827608, -20.95977551465544764 ) ) ;
#11613=CARTESIAN_POINT ( 'NONE',  ( 82.88348280418499314, 63.23117012791774982, -25.51603149568004270 ) ) ;
#11619=CARTESIAN_POINT ( 'NONE',  ( 65.85653452118970108, 79.88098746475269252, -21.59168343458891215 ) ) ;
#11657=CARTESIAN_POINT ( 'NONE',  ( 66.96769116650702358, 79.01678623947613289, -2.861952279419488487 ) ) ;
#11683=CARTESIAN_POINT ( 'NONE',  ( 79.35860935848843667, 49.49491951135498624, -12.08921526900124732 ) ) ;
#11691=CARTESIAN_POINT ( 'NONE',  ( 81.43927332018711240, 61.73960023225036764, -25.08884268687368646 ) ) ;
#11701=CARTESIAN_POINT ( 'NONE',  ( 54.25045881837945672, 77.99799617759832415, -11.96483503560339301 ) ) ;
#11721=CARTESIAN_POINT ( 'NONE',  ( 81.17986817265170885, 58.60139082422833212, -23.83753921867890924 ) ) ;
#11742=( NAMED_UNIT ( * ) SI_UNIT ( $, .STERADIAN. ) SOLID_ANGLE_UNIT ( ) );
#11763=CARTESIAN_POINT ( 'NONE',  ( 62.83629031002387677, 78.04075569348968600, -12.39075692183127941 ) ) ;
#11789=CARTESIAN_POINT ( 'NONE',  ( 78.17606435269406973, 52.48910905489428558, -8.931864344943981848 ) ) ;
#11796=CARTESIAN_POINT ( 'NONE',  ( 75.32572401052811983, 52.39125122145336633, -9.316704993171171623 ) ) ;
#11823=CARTESIAN_POINT ( 'NONE',  ( 82.60978052030384333, 59.60460182822771458, -24.77599324758051580 ) ) ;
#11832=DIRECTION ( 'NONE',  ( 0.8660254037844361541, 0.5000000000000044409, 0.000000000000000000 ) ) ;
#11842=ORIENTED_EDGE ( 'NONE', *, *, #3142, .F. ) ;
#11844=CARTESIAN_POINT ( 'NONE',  ( 81.54430079493101857, 62.01789667144628027, 0.1610543161642296051 ) ) ;
#11866=CARTESIAN_POINT ( 'NONE',  ( 62.79164080153381633, 78.06686219698755735, -12.37752595184878679 ) ) ;
#11937=CARTESIAN_POINT ( 'NONE',  ( 80.80276550169267580, 60.34984310387103790, -24.64969702106051841 ) ) ;
#11976=CARTESIAN_POINT ( 'NONE',  ( 58.58539060705097512, 85.49268159961985702, -12.94168883615076560 ) ) ;
#12004=CARTESIAN_POINT ( 'NONE',  ( 78.99950773051419617, 54.06482698700312284, -5.421535311907622834 ) ) ;
#12010=CARTESIAN_POINT ( 'NONE',  ( 75.54027896286939381, 52.67632256924044754, -8.347856068937160146 ) ) ;
#12034=CARTESIAN_POINT ( 'NONE',  ( 74.47592707218369412, 73.05594451708931558, -24.62326922035613208 ) ) ;
#12039=CARTESIAN_POINT ( 'NONE',  ( 80.21267746518212505, 56.48438466791053258, -22.35508466618705015 ) ) ;
#12058=CARTESIAN_POINT ( 'NONE',  ( 80.22357501274980507, 59.31776527496312923, -0.7804667811256712495 ) ) ;
#12061=DIRECTION ( 'NONE',  ( 0.000000000000000000, 0.6847449705900804373, -0.7287827695902187042 ) ) ;
#12063=AXIS2_PLACEMENT_3D ( 'NONE', #17814, #6873, #14967 ) ;
#12076=CARTESIAN_POINT ( 'NONE',  ( 62.41741185223617805, 78.28105863300197598, -15.10370911918632331 ) ) ;
#12102=CARTESIAN_POINT ( 'NONE',  ( 76.86472363869455648, 54.45620830782070954, -4.878812238591026862 ) ) ;
#12110=CARTESIAN_POINT ( 'NONE',  ( 75.08392619713679039, 52.07086927207439686, -10.97824920096100065 ) ) ;
#12135=CARTESIAN_POINT ( 'NONE',  ( 68.52857421331229659, 77.79673560728132031, -22.80503257933564853 ) ) ;
#12142=CARTESIAN_POINT ( 'NONE',  ( 82.89519626194027069, 61.38757715954039185, -25.23100993346370302 ) ) ;
#12178=CARTESIAN_POINT ( 'NONE',  ( 54.25075523830079760, 77.99786835657231165, -12.14770500197372627 ) ) ;
#12197=CARTESIAN_POINT ( 'NONE',  ( 61.55523633728010680, 134.3395726428436774, -12.50000000000000000 ) ) ;
#12273=ORIENTED_EDGE ( 'NONE', *, *, #4632, .F. ) ;
#12324=CARTESIAN_POINT ( 'NONE',  ( 76.18374514106935180, 68.28054226513678771, 0.08292959599182991859 ) ) ;
#12344=FACE_OUTER_BOUND ( 'NONE', #19697, .T. ) ;
#12377=CARTESIAN_POINT ( 'NONE',  ( 79.36047190431935405, 49.50000000000002842, -12.49999999998710898 ) ) ;
#12430=CARTESIAN_POINT ( 'NONE',  ( 81.96650144582014264, 64.62052529102815868, 0.4991931981429228449 ) ) ;
#12437=ORIENTED_EDGE ( 'NONE', *, *, #14894, .F. ) ;
#12512=CARTESIAN_POINT ( 'NONE',  ( 81.11443760607866693, 65.90576556446161760, -25.47662540745488613 ) ) ;
#12525=CARTESIAN_POINT ( 'NONE',  ( 79.68127019285799406, 68.50330513000922394, 0.4783565974505511464 ) ) ;
#12541=CARTESIAN_POINT ( 'NONE',  ( 63.47128125378750951, 81.72905832825074413, -20.14264400969036828 ) ) ;
#12600=ORIENTED_EDGE ( 'NONE', *, *, #61, .T. ) ;
#12631=CARTESIAN_POINT ( 'NONE',  ( 82.32960224396195770, 63.12647830926369608, 0.3677484777158103735 ) ) ;
#12633=VECTOR ( 'NONE', #4728, 1000.000000000000114 ) ;
#12686=EDGE_CURVE ( 'NONE', #2714, #5808, #13346, .T. ) ;
#12722=CARTESIAN_POINT ( 'NONE',  ( 77.26841646078648296, 67.71923746528655386, -25.22008900393981179 ) ) ;
#12728=CARTESIAN_POINT ( 'NONE',  ( 81.11374900390920573, 66.94010251607396356, 0.6002589370414413983 ) ) ;
#12756=CARTESIAN_POINT ( 'NONE',  ( 76.75377061793378175, 71.15635013821236043, 0.07322384800663080118 ) ) ;
#12808=ORIENTED_EDGE ( 'NONE', *, *, #9633, .F. ) ;
#12836=CARTESIAN_POINT ( 'NONE',  ( 66.21520157169484833, 72.86177730317662338, -2.126289421695329640 ) ) ;
#12862=CARTESIAN_POINT ( 'NONE',  ( 81.23367086208386922, 54.81645704650414785, -2.629400372493356119 ) ) ;
#12877=VERTEX_POINT ( 'NONE', #13985 ) ;
#12883=AXIS2_PLACEMENT_3D ( 'NONE', #6365, #1202, #7654 ) ;
#12905=DIRECTION ( 'NONE',  ( -0.8660254037844362651, -0.5000000000000042188, 0.000000000000000000 ) ) ;
#12909=AXIS2_PLACEMENT_3D ( 'NONE', #19983, #1975, #11832 ) ;
#12930=CIRCLE ( 'NONE', #59, 12.99999999999999822 ) ;
#12943=CARTESIAN_POINT ( 'NONE',  ( 65.99961509271065552, 79.76980348214863170, -3.334180729184369696 ) ) ;
#12946=CARTESIAN_POINT ( 'NONE',  ( 31.00000000000000711, 65.00000000000000000, -22.49999999999999645 ) ) ;
#12971=CARTESIAN_POINT ( 'NONE',  ( 82.41701720340896031, 64.90144913130031057, 0.6268774674042598694 ) ) ;
#12973=CARTESIAN_POINT ( 'NONE',  ( 75.04800910938280367, 52.02334688640443972, -11.56191590910611389 ) ) ;
#12977=UNCERTAINTY_MEASURE_WITH_UNIT (LENGTH_MEASURE( 1.000000000000000082E-05 ), #9407, 'distance_accuracy_value', 'NONE');
#12986=CARTESIAN_POINT ( 'NONE',  ( 56.32485119810130669, 77.11604862365510371, -17.22740159993880482 ) ) ;
#13006=CARTESIAN_POINT ( 'NONE',  ( 69.47824080215001175, 71.42279538029322339, -23.81892892278162677 ) ) ;
#13046=CARTESIAN_POINT ( 'NONE',  ( 64.14641058282846586, 81.20660516694680098, -4.421514697542901828 ) ) ;
#13071=CARTESIAN_POINT ( 'NONE',  ( 58.87500628332524855, 85.27019789096429747, -10.51825745130593859 ) ) ;
#13074=CARTESIAN_POINT ( 'NONE',  ( 79.63536887191790470, 50.25278888007263589, -8.464988250521633617 ) ) ;
#13078=EDGE_LOOP ( 'NONE', ( #11004, #16390, #11842, #16805 ) ) ;
#13082=CIRCLE ( 'NONE', #12063, 11.50000000000002665 ) ;
#13090=CARTESIAN_POINT ( 'NONE',  ( 54.44419410798747094, 77.91572085402148673, -11.00332497362847661 ) ) ;
#13099=VERTEX_POINT ( 'NONE', #10998 ) ;
#13125=CARTESIAN_POINT ( 'NONE',  ( 86.00000000000000000, 65.00000000000000000, -25.50000000000000000 ) ) ;
#13145=CARTESIAN_POINT ( 'NONE',  ( 54.66261616134040935, 77.82294148670094103, -10.34700014260098477 ) ) ;
#13156=VERTEX_POINT ( 'NONE', #8213 ) ;
#13168=ORIENTED_EDGE ( 'NONE', *, *, #2573, .T. ) ;
#13172=CARTESIAN_POINT ( 'NONE',  ( 81.75707366940763166, 56.44708661917523074, -1.582674401186259239 ) ) ;
#13174=CARTESIAN_POINT ( 'NONE',  ( 79.54042647876013916, 49.99209421428520272, -9.220066387385379869 ) ) ;
#13193=CARTESIAN_POINT ( 'NONE',  ( 59.95697519919451679, 75.56535091951175787, -20.09837848646736802 ) ) ;
#13227=CIRCLE ( 'NONE', #7790, 11.50000000000002665 ) ;
#13252=CARTESIAN_POINT ( 'NONE',  ( 56.88554678750333693, 76.87726758071406152, -7.198550218680361823 ) ) ;
#13279=CARTESIAN_POINT ( 'NONE',  ( 79.37883709688843226, 49.55007393176662589, -13.67411419991173283 ) ) ;
#13287=CARTESIAN_POINT ( 'NONE',  ( 78.58128847415450480, 56.84536754178166262, -22.64245902371946784 ) ) ;
#13297=CARTESIAN_POINT ( 'NONE',  ( 77.09271508488680524, 67.80735157681689884, 0.1955130872258976915 ) ) ;
#13318=CARTESIAN_POINT ( 'NONE',  ( 80.02873681804580031, 56.10702248625631228, -22.01643817346699450 ) ) ;
#13346=B_SPLINE_CURVE_WITH_KNOTS ( 'NONE', 3,
 ( #1379, #7832, #19388, #11436, #3, #1586, #11238, #14331, #14538, #4756, #20763, #12722, #15811, #3071, #19185, #6538, #16021, #14430, #6333, #9725 ),
 .UNSPECIFIED., .F., .F.,
 ( 4, 2, 2, 2, 2, 2, 2, 2, 2, 4 ),
 ( 0.09234794266491903880, 0.09522624378769738163, 0.09810454491047572445, 0.1038611471560324101, 0.1067394482788107390, 0.1096177494015890680, 0.1124960505243673969, 0.1139352010857565822, 0.1146547763664511471, 0.1153743516471457259 ),
 .UNSPECIFIED. ) ;
#13355=CARTESIAN_POINT ( 'NONE',  ( 54.59993483903557632, 77.84956924708853876, -14.48805868377909611 ) ) ;
#13374=ORIENTED_EDGE ( 'NONE', *, *, #12686, .F. ) ;
#13378=CARTESIAN_POINT ( 'NONE',  ( 79.36280640676876885, 49.50636784572148485, -13.14917256677527746 ) ) ;
#13397=CARTESIAN_POINT ( 'NONE',  ( 60.75500010343246515, 75.22326679826591089, -20.54849183009933711 ) ) ;
#13418=CARTESIAN_POINT ( 'NONE',  ( 80.59332237824474987, 57.28794717993011432, -22.99282313644232900 ) ) ;
#13460=CARTESIAN_POINT ( 'NONE',  ( 56.17290541411050953, 77.18071550550122595, -17.04775252395419116 ) ) ;
#13472=PRODUCT_DEFINITION_SHAPE ( 'NONE', 'NONE',  #11582 ) ;
#13485=CARTESIAN_POINT ( 'NONE',  ( 80.72059958497800380, 57.56183285562485707, -1.811819122334661358 ) ) ;
#13489=CARTESIAN_POINT ( 'NONE',  ( 80.42500778927126248, 52.45643482355421128, -4.799589912607079789 ) ) ;
#13497=CARTESIAN_POINT ( 'NONE',  ( 81.68143887139700610, 63.75701689938041739, -25.44160877821855848 ) ) ;
#13511=DIRECTION ( 'NONE',  ( 0.8660254037844360431, 0.5000000000000044409, 0.000000000000000000 ) ) ;
#13520=CARTESIAN_POINT ( 'NONE',  ( 77.44988535257863305, 70.55865560739972864, -25.18692877124620466 ) ) ;
#13523=CARTESIAN_POINT ( 'NONE',  ( 81.45340819612970051, 61.78983808953367429, -25.10003246456431825 ) ) ;
#13545=CARTESIAN_POINT ( 'NONE',  ( 78.25962792613263730, 56.38842605307239353, -2.753243699805369982 ) ) ;
#13547=DIRECTION ( 'NONE',  ( -0.5000000000000045519, 0.8660254037844360431, 0.000000000000000000 ) ) ;
#13565=CARTESIAN_POINT ( 'NONE',  ( 62.88012315395636875, 78.01512619438163654, -12.57944489567368329 ) ) ;
#13567=ORIENTED_EDGE ( 'NONE', *, *, #2684, .F. ) ;
#13576=DIRECTION ( 'NONE',  ( 1.000000000000000000, -0.000000000000000000, -0.000000000000000000 ) ) ;
#13594=CARTESIAN_POINT ( 'NONE',  ( 81.85367731271401226, 60.34691469923900797, -0.3446091499246847212 ) ) ;
#13599=CARTESIAN_POINT ( 'NONE',  ( 80.06776404988029583, 51.44734343012801503, -6.071549608444867907 ) ) ;
#13602=CIRCLE ( 'NONE', #7483, 13.50000000000000178 ) ;
#13606=CARTESIAN_POINT ( 'NONE',  ( 77.04324694534321338, 54.69866214318452080, -20.45431430911883908 ) ) ;
#13635=CARTESIAN_POINT ( 'NONE',  ( 82.20788507225606168, 63.93871732008117448, -25.46035155396378968 ) ) ;
#13636=CARTESIAN_POINT ( 'NONE',  ( 59.05164960708168564, 85.13446652039156959, -14.98897224784199800 ) ) ;
#13652=CARTESIAN_POINT ( 'NONE',  ( 61.57468973143931379, 74.87077495648827608, -20.95977551465544764 ) ) ;
#13672=CARTESIAN_POINT ( 'NONE',  ( 62.26115743202674224, 78.37397343634121682, -14.48362007552005437 ) ) ;
#13706=CARTESIAN_POINT ( 'NONE',  ( 79.58925804534456461, 58.33401430123417697, -23.67724775046685437 ) ) ;
#13735=CARTESIAN_POINT ( 'NONE',  ( 79.67828149300846974, 55.39867050251828573, -21.30364596931944376 ) ) ;
#13756=DIRECTION ( 'NONE',  ( -0.5000000000000045519, 0.8660254037844360431, 0.000000000000000000 ) ) ;
#13774=CARTESIAN_POINT ( 'NONE',  ( 60.49916866905066115, 75.33328221149844239, -20.42012703083461389 ) ) ;
#13780=ORIENTED_EDGE ( 'NONE', *, *, #10639, .T. ) ;
#13804=CARTESIAN_POINT ( 'NONE',  ( 77.55491039835763445, 55.40237803623692514, -3.717510863212275307 ) ) ;
#13814=PLANE ( 'NONE',  #20490 ) ;
#13832=ORIENTED_EDGE ( 'NONE', *, *, #490, .T. ) ;
#13890=LINE ( 'NONE', #17172, #15853 ) ;
#13918=DIRECTION ( 'NONE',  ( -1.000000000000000000, 0.000000000000000000, 0.000000000000000000 ) ) ;
#13940=ORIENTED_EDGE ( 'NONE', *, *, #5872, .T. ) ;
#13969=AXIS2_PLACEMENT_3D ( 'NONE', #1661, #7901, #12905 ) ;
#13985=CARTESIAN_POINT ( 'NONE',  ( 31.00000000000000711, 65.00000000000000000, -2.500000000000005773 ) ) ;
#14018=CARTESIAN_POINT ( 'NONE',  ( 80.76021944741209779, 65.35629346140643747, 0.4967719932253782389 ) ) ;
#14046=ORIENTED_EDGE ( 'NONE', *, *, #2816, .F. ) ;
#14118=CARTESIAN_POINT ( 'NONE',  ( 80.60041742765380945, 65.51180379921632380, -25.49148684086367211 ) ) ;
#14130=CARTESIAN_POINT ( 'NONE',  ( 79.87047281314329439, 67.12885141646589204, 0.3411143157775017309 ) ) ;
#14144=DIRECTION ( 'NONE',  ( 0.8660254037844359321, 0.5000000000000046629, 0.000000000000000000 ) ) ;
#14164=CARTESIAN_POINT ( 'NONE',  ( 66.35003277998524140, 79.49709411292175787, -21.83015642861430550 ) ) ;
#14203=ORIENTED_EDGE ( 'NONE', *, *, #4632, .T. ) ;
#14223=FACE_OUTER_BOUND ( 'NONE', #9556, .T. ) ;
#14234=CARTESIAN_POINT ( 'NONE',  ( 80.65040410709035257, 67.47975763685462880, 0.5668321014029960025 ) ) ;
#14260=DIRECTION ( 'NONE',  ( 0.5000000000000041078, -0.8660254037844362651, 0.000000000000000000 ) ) ;
#14308=VERTEX_POINT ( 'NONE', #8106 ) ;
#14310=DIRECTION ( 'NONE',  ( 1.000000000000000000, -0.000000000000000000, -0.000000000000000000 ) ) ;
#14331=CARTESIAN_POINT ( 'NONE',  ( 72.24503483210654053, 70.17032258213592399, -24.43510331009084524 ) ) ;
#14338=CARTESIAN_POINT ( 'NONE',  ( 81.70593518416212930, 63.65981237297968676, 0.4334013042838535390 ) ) ;
#14367=CARTESIAN_POINT ( 'NONE',  ( 60.59842726415620717, 83.94481412498421946, -7.461880171922929961 ) ) ;
#14430=CARTESIAN_POINT ( 'NONE',  ( 80.75261313425734500, 65.35990508136943333, -25.49604157242841396 ) ) ;
#14439=CARTESIAN_POINT ( 'NONE',  ( 78.48791029091835014, 67.03256333895615171, 0.3448344096533276781 ) ) ;
#14448=PRODUCT_CONTEXT ( 'NONE', #14637, 'mechanical' ) ;
#14468=CARTESIAN_POINT ( 'NONE',  ( 82.39092640778034138, 58.62218493319811330, -0.5469516794101250134 ) ) ;
#14533=( NAMED_UNIT ( * ) SI_UNIT ( $, .STERADIAN. ) SOLID_ANGLE_UNIT ( ) );
#14538=CARTESIAN_POINT ( 'NONE',  ( 73.08722033050757716, 69.78136637326532821, -24.59619082723051164 ) ) ;
#14544=CARTESIAN_POINT ( 'NONE',  ( 59.14831028279606073, 75.91136029574231259, -5.422152313826261505 ) ) ;
#14580=VERTEX_POINT ( 'NONE', #10752 ) ;
#14587=CARTESIAN_POINT ( 'NONE',  ( 55.44059175264857231, 77.49228655561917378, -16.12265240795897725 ) ) ;
#14598=ORIENTED_EDGE ( 'NONE', *, *, #16034, .F. ) ;
#14610=CARTESIAN_POINT ( 'NONE',  ( 68.76802220417130229, 77.60947533363440698, -22.90979173856745277 ) ) ;
#14637=APPLICATION_CONTEXT ( 'automotive_design' ) ;
#14655=CARTESIAN_POINT ( 'NONE',  ( 63.92888185421814740, 73.85612640264653805, -2.961109148988000594 ) ) ;
#14667=DIRECTION ( 'NONE',  ( 0.000000000000000000, 0.000000000000000000, -1.000000000000000000 ) ) ;
#14680=CARTESIAN_POINT ( 'NONE',  ( 64.01501096541383617, 81.30857500227412515, -4.496114496788966797 ) ) ;
#14683=CARTESIAN_POINT ( 'NONE',  ( 75.50233069471819647, 52.62586201590558943, -8.506500717077631890 ) ) ;
#14695=CARTESIAN_POINT ( 'NONE',  ( 54.59239912755987945, 77.85276913609830274, -10.53475018185270251 ) ) ;
#14755=CARTESIAN_POINT ( 'NONE',  ( 62.39943480050086322, 78.29596884051593975, -12.34141208372355258 ) ) ;
#14781=CARTESIAN_POINT ( 'NONE',  ( 82.84955722239773479, 63.45971040577538957, 0.5391910165619532291 ) ) ;
#14783=CARTESIAN_POINT ( 'NONE',  ( 78.44171698552800365, 52.99314787609267086, -17.60414262153716791 ) ) ;
#14785=ORIENTED_EDGE ( 'NONE', *, *, #3841, .T. ) ;
#14798=CARTESIAN_POINT ( 'NONE',  ( 80.18983717961930324, 65.86547942624545726, 0.4720184283333879183 ) ) ;
#14819=CARTESIAN_POINT ( 'NONE',  ( 79.37802773247075550, 66.47170366897312022, -25.42092142087688700 ) ) ;
#14849=VECTOR ( 'NONE', #7792, 1000.000000000000000 ) ;
#14856=ADVANCED_FACE ( 'NONE', ( #875, #7325 ), #13814, .T. ) ;
#14858=CARTESIAN_POINT ( 'NONE',  ( 69.07465262935465944, 74.30594400923098419, -3.091493055308389248 ) ) ;
#14885=CARTESIAN_POINT ( 'NONE',  ( 79.59702692428714954, 50.14740214866447587, -16.24970959789619940 ) ) ;
#14893=CARTESIAN_POINT ( 'NONE',  ( 76.11375628839972762, 53.44186132163859071, -6.514818636118950401 ) ) ;
#14894=EDGE_CURVE ( 'NONE', #11548, #8298, #3230, .T. ) ;
#14900=CARTESIAN_POINT ( 'NONE',  ( 64.97908659311265467, 73.40006927592642683, -2.567007515994158773 ) ) ;
#14912=CARTESIAN_POINT ( 'NONE',  ( 72.22890356904881060, 74.87903105603933795, -24.07778875527023743 ) ) ;
#14916=CARTESIAN_POINT ( 'NONE',  ( 77.89229590160842065, 55.87094247655682011, -21.76811895496497584 ) ) ;
#14959=CARTESIAN_POINT ( 'NONE',  ( 59.12621987370580001, 85.07716061577534106, -9.825189264790521904 ) ) ;
#14967=DIRECTION ( 'NONE',  ( 0.8660254037844359321, 0.5000000000000046629, 0.000000000000000000 ) ) ;
#14995=CARTESIAN_POINT ( 'NONE',  ( 78.02789439511529679, 52.20891951634391859, -14.88908151311502870 ) ) ;
#15002=CARTESIAN_POINT ( 'NONE',  ( 77.63095968975100902, 55.50711545842607819, -21.40358471902519000 ) ) ;
#15011=CARTESIAN_POINT ( 'NONE',  ( 55.76083050669604546, 77.35608213855016402, -8.438634470110439878 ) ) ;
#15017=DIRECTION ( 'NONE',  ( 0.5000000000000045519, -0.8660254037844362651, 0.000000000000000000 ) ) ;
#15026=CARTESIAN_POINT ( 'NONE',  ( 82.47279574233218113, 58.94507879694565133, -24.57151460914693075 ) ) ;
#15033=CARTESIAN_POINT ( 'NONE',  ( 82.19079093293210292, 61.61208316210709057, -25.05535973731833366 ) ) ;
#15065=FACE_OUTER_BOUND ( 'NONE', #13078, .T. ) ;
#15071=CARTESIAN_POINT ( 'NONE',  ( 59.50745032656949718, 84.78413469058132534, -15.98776567044169994 ) ) ;
#15093=CARTESIAN_POINT ( 'NONE',  ( 79.78989234911249184, 55.62452637193754867, -3.470983589548607640 ) ) ;
#15096=CARTESIAN_POINT ( 'NONE',  ( 79.19901074457860091, 54.45260783255401549, -20.14565730162479085 ) ) ;
#15102=CARTESIAN_POINT ( 'NONE',  ( 78.05328906524978549, 56.09831538232894843, -3.025823995327162841 ) ) ;
#15129=CARTESIAN_POINT ( 'NONE',  ( 82.83006403966726339, 60.80631076346477926, -25.10535189848144455 ) ) ;
#15133=ADVANCED_FACE ( 'NONE', ( #14223 ), #17651, .F. ) ;
#15134=CARTESIAN_POINT ( 'NONE',  ( 79.20517720625409197, 57.75691248093230001, -23.30626794376461319 ) ) ;
#15176=CARTESIAN_POINT ( 'NONE',  ( 59.16309583933880845, 85.04882181297647037, -15.26077928376918358 ) ) ;
#15209=CARTESIAN_POINT ( 'NONE',  ( 76.25855100882986903, 53.63624723668596772, -18.84667540378509898 ) ) ;
#15238=CARTESIAN_POINT ( 'NONE',  ( 77.17349984701002086, 54.87731286059718627, -20.67167348712315444 ) ) ;
#15239=CARTESIAN_POINT ( 'NONE',  ( 60.23610500267373169, 84.22369677626844009, -17.09587939145292523 ) ) ;
#15279=CARTESIAN_POINT ( 'NONE',  ( 62.22363694231594167, 78.39636059616459818, -14.27859498331829080 ) ) ;
#15293=VECTOR ( 'NONE', #5048, 1000.000000000000000 ) ;
#15317=CARTESIAN_POINT ( 'NONE',  ( 81.31407792830592030, 61.42543535009416900, -25.00296011795888518 ) ) ;
#15341=CARTESIAN_POINT ( 'NONE',  ( 81.34596348373698049, 55.15737503394385755, -22.61349628177035243 ) ) ;
#15343=CYLINDRICAL_SURFACE ( 'NONE', #10633, 13.50000000000000711 ) ;
#15345=CARTESIAN_POINT ( 'NONE',  ( 81.19763523304686714, 64.84546557366820707, -25.50103675175597573 ) ) ;
#15346=CARTESIAN_POINT ( 'NONE',  ( 58.69853696180994262, 85.40577002866142209, -13.78609211422347869 ) ) ;
#15374=CARTESIAN_POINT ( 'NONE',  ( 49.86389338619021316, 127.5895726428436205, -12.50000000000000000 ) ) ;
#15386=CARTESIAN_POINT ( 'NONE',  ( 63.20289482801889847, 77.81544268501482975, -16.80222038511762506 ) ) ;
#15394=LINE ( 'NONE', #10257, #1951 ) ;
#15408=CARTESIAN_POINT ( 'NONE',  ( 81.67521804894028037, 59.84799745248609071, -0.5475991497997765300 ) ) ;
#15427=CARTESIAN_POINT ( 'NONE',  ( 38.17255043510031953, 120.8395726428435637, -12.49999999999999822 ) ) ;
#15438=CARTESIAN_POINT ( 'NONE',  ( 65.63317740310760939, 80.05417074498873831, -21.46107424520661411 ) ) ;
#15451=CLOSED_SHELL ( 'NONE', ( #10590, #4195, #1764, #6828, #7726, #9885, #3768, #18434, #14856, #10346, #6667, #6550, #15133, #3929 ) ) ;
#15499=EDGE_CURVE ( 'NONE', #5375, #13099, #13082, .T. ) ;
#15609=CARTESIAN_POINT ( 'NONE',  ( 79.56209656442725020, 66.33713882184865440, 0.4323996719432884883 ) ) ;
#15615=CARTESIAN_POINT ( 'NONE',  ( 80.82197242644828350, 53.59722411448979074, -3.626216797365716005 ) ) ;
#15636=ORIENTED_EDGE ( 'NONE', *, *, #8968, .T. ) ;
#15719=CARTESIAN_POINT ( 'NONE',  ( 74.25247827671769585, 71.10552778957739406, -0.9041564858560480200 ) ) ;
#15725=SHAPE_DEFINITION_REPRESENTATION ( #13472, #16277 ) ;
#15751=CARTESIAN_POINT ( 'NONE',  ( 67.79769812808454788, 78.36839442147740442, -22.50225811741774606 ) ) ;
#15811=CARTESIAN_POINT ( 'NONE',  ( 78.09128061238048701, 67.27484481498704838, -25.30919057591654209 ) ) ;
#15815=PLANE ( 'NONE',  #5813 ) ;
#15818=CARTESIAN_POINT ( 'NONE',  ( 80.06760114659269334, 65.96496744433481751, 0.4654826109615978758 ) ) ;
#15829=CARTESIAN_POINT ( 'NONE',  ( 59.70164726310041203, 84.63482219402854412, -16.31058207722989195 ) ) ;
#15840=CARTESIAN_POINT ( 'NONE',  ( 86.00000000000000000, 65.00000000000000000, -12.50000000000000000 ) ) ;
#15853=VECTOR ( 'NONE', #2654, 1000.000000000000227 ) ;
#15903=CARTESIAN_POINT ( 'NONE',  ( 0.000000000000000000, 0.000000000000000000, 0.000000000000000000 ) ) ;
#15918=CARTESIAN_POINT ( 'NONE',  ( 69.70673644162950211, 71.32081881487549424, -1.123846180645351023 ) ) ;
#15944=CARTESIAN_POINT ( 'NONE',  ( 58.80511404976427769, 85.32389451869947550, -10.75888619813460423 ) ) ;
#15952=AXIS2_PLACEMENT_3D ( 'NONE', #4328, #14310, #17257 ) ;
#16021=CARTESIAN_POINT ( 'NONE',  ( 80.40479875449686631, 65.68600401853653636, -25.48291287448371278 ) ) ;
#16029=CARTESIAN_POINT ( 'NONE',  ( 81.45372947444067790, 64.43233774075389420, 0.4901336013121079804 ) ) ;
#16034=EDGE_CURVE ( 'NONE', #7029, #14580, #19837, .T. ) ;
#16055=CARTESIAN_POINT ( 'NONE',  ( 77.50589888911159164, 70.51031857425567750, 0.1958985337333214449 ) ) ;
#16090=CARTESIAN_POINT ( 'NONE',  ( 38.17255043510031953, 120.8395726428435637, -12.49999999999999822 ) ) ;
#16099=EDGE_LOOP ( 'NONE', ( #20748, #14785, #17392, #6580, #13780, #19522, #1940 ) ) ;
#16126=CARTESIAN_POINT ( 'NONE',  ( 62.63374148850010670, 78.15280783560238831, -9.335207922937284408 ) ) ;
#16169=CARTESIAN_POINT ( 'NONE',  ( 76.66199489384241872, 68.03321850950067073, 0.1432382234697572587 ) ) ;
#16176=ORIENTED_EDGE ( 'NONE', *, *, #17676, .F. ) ;
#16188=CARTESIAN_POINT ( 'NONE',  ( 70.88961965102326701, 73.20066112274578529, -22.81645270491783251 ) ) ;
#16201=ORIENTED_EDGE ( 'NONE', *, *, #8968, .F. ) ;
#16218=CARTESIAN_POINT ( 'NONE',  ( 55.93063010822693570, 77.28382646649683352, -8.238606096522689271 ) ) ;
#16243=CARTESIAN_POINT ( 'NONE',  ( 58.57586221349182409, 85.50000000000065370, -12.24792819076230366 ) ) ;
#16245=CARTESIAN_POINT ( 'NONE',  ( 79.46180180641687230, 49.77667888093298387, -9.984653723550882987 ) ) ;
#16246=APPLICATION_CONTEXT ( 'automotive_design' ) ;
#16261=CARTESIAN_POINT ( 'NONE',  ( 57.73559688320084149, 76.51496841747558619, -6.433815121522095559 ) ) ;
#16277=SHAPE_REPRESENTATION ( '60-Degree Angle Clamping Handle', ( #18233 ), #16874 ) ;
#16285=CARTESIAN_POINT ( 'NONE',  ( 76.78232915647551238, 69.44169262812657450, -24.77272969115283274 ) ) ;
#16329=CARTESIAN_POINT ( 'NONE',  ( 68.95169418938438355, 77.46545255404963370, -2.018454592414399951 ) ) ;
#16354=CARTESIAN_POINT ( 'NONE',  ( 68.41618888151715794, 77.88480544091760294, -2.239802524522644944 ) ) ;
#16356=CARTESIAN_POINT ( 'NONE',  ( 79.66622197694607621, 50.33767513494625945, -16.74958941344072016 ) ) ;
#16370=CARTESIAN_POINT ( 'NONE',  ( 55.07002310602048567, 77.64981942332057940, -15.50454273085438928 ) ) ;
#16390=ORIENTED_EDGE ( 'NONE', *, *, #2684, .T. ) ;
#16392=CARTESIAN_POINT ( 'NONE',  ( 74.22444910852603073, 69.25129922422347306, -24.80018073758580854 ) ) ;
#16427=ORIENTED_EDGE ( 'NONE', *, *, #3841, .F. ) ;
#16428=CARTESIAN_POINT ( 'NONE',  ( 54.56775351867148771, 77.86323848837362505, -10.60172925492977214 ) ) ;
#16449=CARTESIAN_POINT ( 'NONE',  ( 75.55536774603304195, 52.69641891097137432, -16.70586935774736759 ) ) ;
#16466=CARTESIAN_POINT ( 'NONE',  ( 80.37830472862586362, 65.70931303850179006, 0.4817205432224337947 ) ) ;
#16481=CARTESIAN_POINT ( 'NONE',  ( 81.47374219290158237, 55.54988310573300936, -22.87663793174895943 ) ) ;
#16486=CARTESIAN_POINT ( 'NONE',  ( 62.64765726746416874, 74.40936579681903140, -21.49814275265928742 ) ) ;
#16491=DIRECTION ( 'NONE',  ( 0.000000000000000000, 0.000000000000000000, -1.000000000000000000 ) ) ;
#16528=CARTESIAN_POINT ( 'NONE',  ( 59.60168565680741892, 84.71166588009855047, -8.872864206773611429 ) ) ;
#16558=CARTESIAN_POINT ( 'NONE',  ( 78.13892160451581503, 52.41879779276553819, -15.80834409985953926 ) ) ;
#16573=CARTESIAN_POINT ( 'NONE',  ( 57.68399219382784793, 76.53693708094122883, -18.53323648005439139 ) ) ;
#16590=CARTESIAN_POINT ( 'NONE',  ( 82.31356959450070576, 63.34177109540507189, -25.39725247914766726 ) ) ;
#16621=EDGE_LOOP ( 'NONE', ( #4946, #4546, #13940, #6795, #10356 ) ) ;
#16634=CARTESIAN_POINT ( 'NONE',  ( 54.51375964220392234, 77.88617331000196486, -14.23577307808955972 ) ) ;
#16663=CARTESIAN_POINT ( 'NONE',  ( 81.55608559449183304, 62.10651918161714491, 0.1764946495667281956 ) ) ;
#16666=CARTESIAN_POINT ( 'NONE',  ( 79.86683865086524747, 50.89072876157985803, -6.984412221717008151 ) ) ;
#16673=CARTESIAN_POINT ( 'NONE',  ( 75.15809445383052889, 52.16896057810638609, -10.30453221435095834 ) ) ;
#16700=CARTESIAN_POINT ( 'NONE',  ( 80.07168963752003776, 51.46048616005985821, -18.93354426913304422 ) ) ;
#16705=CARTESIAN_POINT ( 'NONE',  ( 82.20437289446037710, 57.97282872583890168, -24.17078908960660755 ) ) ;
#16722=CARTESIAN_POINT ( 'NONE',  ( 81.33476212519650517, 64.63473428484439864, 0.4964296018791880538 ) ) ;
#16734=CIRCLE ( 'NONE', #8256, 5.000000000000000000 ) ;
#16740=CARTESIAN_POINT ( 'NONE',  ( 60.40852599701213421, 84.09099035223172791, -17.30637792422236032 ) ) ;
#16748=EDGE_CURVE ( 'NONE', #11548, #17011, #15394, .T. ) ;
#16763=CARTESIAN_POINT ( 'NONE',  ( 81.10655718899693056, 54.43739570253208626, -2.927339837274431922 ) ) ;
#16773=ORIENTED_EDGE ( 'NONE', *, *, #16748, .F. ) ;
#16805=ORIENTED_EDGE ( 'NONE', *, *, #17348, .F. ) ;
#16806=CARTESIAN_POINT ( 'NONE',  ( 81.73373490635979977, 63.06197297317982020, -25.35741583561241086 ) ) ;
#16811=DIRECTION ( 'NONE',  ( 1.000000000000000000, -0.000000000000000000, -0.000000000000000000 ) ) ;
#16827=LINE ( 'NONE', #10231, #9165 ) ;
#16843=CARTESIAN_POINT ( 'NONE',  ( 54.92373153686620668, 77.71199488874673023, -15.23237620472049336 ) ) ;
#16874=( GEOMETRIC_REPRESENTATION_CONTEXT ( 3 ) GLOBAL_UNCERTAINTY_ASSIGNED_CONTEXT ( ( #12977 ) ) GLOBAL_UNIT_ASSIGNED_CONTEXT ( ( #9407, #6226, #14533 ) ) REPRESENTATION_CONTEXT ( 'NONE', 'WORKASPACE' ) );
#16879=CARTESIAN_POINT ( 'NONE',  ( 75.21428198808020227, 52.24336229720762503, -15.09414418353362031 ) ) ;
#16902=CARTESIAN_POINT ( 'NONE',  ( 79.60733510696749704, 50.17557044886655149, -16.34883357536578785 ) ) ;
#16906=CARTESIAN_POINT ( 'NONE',  ( 81.70322370085452235, 65.10829061386586147, -25.50491105577044237 ) ) ;
#16928=DIRECTION ( 'NONE',  ( -0.3505956610260388406, -0.6825246866719044680, -0.6412821021618595463 ) ) ;
#16946=CARTESIAN_POINT ( 'NONE',  ( 61.88036088246662558, 82.95721218253052598, -18.86925204637720555 ) ) ;
#16987=CARTESIAN_POINT ( 'NONE',  ( 75.03586402968051061, 52.00729864744448605, -13.05716366695459918 ) ) ;
#17011=VERTEX_POINT ( 'NONE', #6637 ) ;
#17013=AXIS2_PLACEMENT_3D ( 'NONE', #15374, #7179, #3677 ) ;
#17020=CARTESIAN_POINT ( 'NONE',  ( 81.01504177493372083, 54.16268467661828367, -21.86446114789482920 ) ) ;
#17039=( NAMED_UNIT ( * ) PLANE_ANGLE_UNIT ( ) SI_UNIT ( $, .RADIAN. ) );
#17062=CARTESIAN_POINT ( 'NONE',  ( 56.36150222382281783, 77.10042895211010716, -17.25692959166989837 ) ) ;
#17087=CARTESIAN_POINT ( 'NONE',  ( 81.40012587587739290, 55.32114690216545938, -2.271216619685866522 ) ) ;
#17172=CARTESIAN_POINT ( 'NONE',  ( 95.83809698076872507, 24.95991617951895236, -12.50000000000000000 ) ) ;
#17186=CARTESIAN_POINT ( 'NONE',  ( 81.65190015349629959, 63.92029392008140576, 0.4576250216425485906 ) ) ;
#17208=DIRECTION ( 'NONE',  ( -1.000000000000000000, 0.000000000000000000, 0.000000000000000000 ) ) ;
#17218=PRODUCT_DEFINITION_CONTEXT ( 'detailed design', #16246, 'design' ) ;
#17241=CARTESIAN_POINT ( 'NONE',  ( 80.86682143426207858, 53.72248789457500351, -3.489252184860733408 ) ) ;
#17257=DIRECTION ( 'NONE',  ( 0.000000000000000000, 0.000000000000000000, -1.000000000000000000 ) ) ;
#17288=CARTESIAN_POINT ( 'NONE',  ( 80.41157793103774054, 67.74023943711713969, 0.5468165597092933261 ) ) ;
#17348=EDGE_CURVE ( 'NONE', #19292, #5200, #10876, .T. ) ;
#17386=CARTESIAN_POINT ( 'NONE',  ( 81.61199360759415811, 66.29268519405596294, -25.62653348100026918 ) ) ;
#17392=ORIENTED_EDGE ( 'NONE', *, *, #8782, .T. ) ;
#17397=CARTESIAN_POINT ( 'NONE',  ( 77.91874456701133056, 67.35752264558084335, 0.2884206837271629520 ) ) ;
#17464=FACE_OUTER_BOUND ( 'NONE', #11261, .T. ) ;
#17486=B_SPLINE_CURVE_WITH_KNOTS ( 'NONE', 3,
 ( #609, #13545, #510, #5565, #713, #3667, #12058, #6952, #5353, #2518, #11844, #8963, #18522, #6851, #18306, #3779, #10229, #16722, #19997, #5458 ),
 .UNSPECIFIED., .F., .F.,
 ( 4, 2, 2, 2, 2, 2, 2, 2, 2, 4 ),
 ( 0.03344032305337923255, 0.03481802353568227981, 0.03619572401798533401, 0.03895112498259143546, 0.04032882546489449660, 0.04170652594719755774, 0.04239537618834907790, 0.04308422642950059805, 0.04377307667065211821, 0.04446192691180363837 ),
 .UNSPECIFIED. ) ;
#17492=CARTESIAN_POINT ( 'NONE',  ( 74.88379549237744470, 72.72378982140247672, -24.71895639200489825 ) ) ;
#17503=CARTESIAN_POINT ( 'NONE',  ( 78.15559533904072964, 69.92979238318895341, 0.2890775442667399830 ) ) ;
#17526=CARTESIAN_POINT ( 'NONE',  ( 81.62532777622794811, 56.02584323239422304, -1.826067817236490365 ) ) ;
#17555=EDGE_LOOP ( 'NONE', ( #16427, #1052, #20379, #3567, #19818, #13832, #232 ) ) ;
#17607=CARTESIAN_POINT ( 'NONE',  ( 82.90420097239591257, 63.09545557312737429, 0.5024926129020395038 ) ) ;
#17609=ORIENTED_EDGE ( 'NONE', *, *, #14894, .T. ) ;
#17631=CARTESIAN_POINT ( 'NONE',  ( 59.42304552939003770, 84.84901963477547326, -9.175363098692354669 ) ) ;
#17651=( BOUNDED_SURFACE ( )  B_SPLINE_SURFACE ( 3, 2, ( 
 ( #9896, #167, #6128 ),
 ( #16486, #17883, #11619 ),
 ( #11022, #18081, #9796 ),
 ( #11404, #19552, #14610 ),
 ( #19082, #1969, #6023 ),
 ( #13006, #16188, #4555 ),
 ( #8207, #5029, #11505 ),
 ( #5133, #2867, #17492 ),
 ( #16392, #1657, #20550 ),
 ( #3549, #16285, #8096 ),
 ( #1762, #19449, #10915 ),
 ( #4928, #1865, #3345 ),
 ( #6611, #17984, #3448 ),
 ( #14819, #268, #4452 ),
 ( #6713, #19660, #9991 ),
 ( #14118, #12512, #17386 ),
 ( #690, #800, #7146 ),
 ( #15345, #16906, #3649 ),
 ( #588, #3760, #19971 ),
 ( #8636, #8533, #10535 ),
 ( #2079, #13635, #8846 ),
 ( #5438, #16590, #20087 ),
 ( #16806, #2285, #18503 ),
 ( #10425, #5333, #6931 ),
 ( #18184, #6835, #5652 ),
 ( #13523, #15033, #12142 ),
 ( #2387, #8740, #18604 ),
 ( #18284, #383, #492 ),
 ( #11937, #19766, #11823 ),
 ( #5230, #4078, #10316 ),
 ( #10212, #11721, #16705 ),
 ( #18396, #3975, #2184 ),
 ( #15134, #13418, #5549 ),
 ( #10102, #12039, #19866 ),
 ( #7252, #13318, #20189 ),
 ( #14916, #13735, #17020 ),
 ( #8416, #7041, #3865 ),
 ( #15238, #15096, #10067 ),
 ( #342, #11470, #5196 ),
 ( #6575, #4993, #4899 ),
 ( #3716, #14783, #19420 ),
 ( #8273, #137, #6788 ),
 ( #16449, #11370, #16356 ),
 ( #18048, #16558, #14885 ),
 ( #8491, #19515, #19619 ),
 ( #8598, #14995, #551 ),
 ( #17845, #452, #6678 ),
 ( #3409, #6898, #13279 ),
 ( #19724, #1725, #13378 ),
 ( #18148, #5297, #11683 ),
 ( #12973, #9761, #237 ),
 ( #3615, #11578, #19829 ),
 ( #1829, #3312, #16245 ),
 ( #5096, #8174, #13174 ),
 ( #9957, #2038, #3516 ),
 ( #14683, #11789, #13074 ),
 ( #17946, #18252, #1936 ),
 ( #9861, #10171, #16666 ),
 ( #8383, #2147, #13599 ),
 ( #12102, #12004, #13489 ),
 ( #2249, #973, #5402 ),
 ( #13804, #7109, #15615 ),
 ( #10489, #4259, #2353 ),
 ( #10711, #2464, #18571 ) ),
 .UNSPECIFIED., .F., .F., .F. ) 
 B_SPLINE_SURFACE_WITH_KNOTS ( ( 4, 2, 2, 2, 2, 2, 2, 2, 2, 2, 2, 2, 2, 2, 2, 2, 2, 2, 2, 2, 2, 2, 2, 2, 2, 2, 2, 2, 2, 2, 2, 4 ),
 ( 3, 3 ),
 ( 0.000000000000000000, 0.004303368843509257358, 0.008606737687018514715, 0.01291010653052777207, 0.01721347537403702943, 0.01936515979579165811, 0.02151684421754628679, 0.02366852863930091547, 0.02474437085017822807, 0.02582021306105554415, 0.02689605527193286022, 0.02797189748281017282, 0.02904773969368748543, 0.03012358190456480150, 0.03227526632631942671, 0.03442695074807405886, 0.03657863516982869101, 0.03873031959158331622, 0.04088200401333794143, 0.04303368843509257358, 0.04733705727860183093, 0.04841289948947914701, 0.04948874170035645614, 0.05164042612211108829, 0.05379211054386572044, 0.05594379496562034565, 0.05809547938737497086, 0.05917132159825228693, 0.06024716380912960301, 0.06455053265263885343, 0.06670221707439348557, 0.06885390149614811772 ),
 ( 0.000000000000000000, 1.000000000000000000 ),
 .UNSPECIFIED. ) 
 GEOMETRIC_REPRESENTATION_ITEM ( )  RATIONAL_B_SPLINE_SURFACE ( (
 ( 1.000000000000000000, 0.7477234448260038358, 1.000000000000000000),
 ( 1.000000000000000000, 0.7740357663989568815, 1.000000000000000000),
 ( 1.000000000000000000, 0.7979944444720340480, 1.000000000000000000),
 ( 1.000000000000000000, 0.8415418573160285964, 1.000000000000000000),
 ( 1.000000000000000000, 0.8611354141022936615, 1.000000000000000000),
 ( 1.000000000000000000, 0.8962784209894617549, 1.000000000000000000),
 ( 1.000000000000000000, 0.9118336320813347218, 1.000000000000000000),
 ( 1.000000000000000000, 0.9390903228898979105, 1.000000000000000000),
 ( 1.000000000000000000, 0.9507059349589174202, 1.000000000000000000),
 ( 1.000000000000000000, 0.9652792442033365505, 1.000000000000000000),
 ( 1.000000000000000000, 0.9696658626168446204, 1.000000000000000000),
 ( 1.000000000000000000, 0.9774477440020008512, 1.000000000000000000),
 ( 1.000000000000000000, 0.9808482499402014776, 1.000000000000000000),
 ( 1.000000000000000000, 0.9866388090191381410, 1.000000000000000000),
 ( 1.000000000000000000, 0.9890362374316506999, 1.000000000000000000),
 ( 1.000000000000000000, 0.9917478669874124630, 1.000000000000000000),
 ( 1.000000000000000000, 0.9925034521094587836, 1.000000000000000000),
 ( 1.000000000000000000, 0.9936052247524241876, 1.000000000000000000),
 ( 1.000000000000000000, 0.9939601189669974302, 1.000000000000000000),
 ( 1.000000000000000000, 0.9942187593714609806, 1.000000000000000000),
 ( 1.000000000000000000, 0.9941154017096719420, 1.000000000000000000),
 ( 1.000000000000000000, 0.9934872688014458886, 1.000000000000000000),
 ( 1.000000000000000000, 0.9929544046041767213, 1.000000000000000000),
 ( 1.000000000000000000, 0.9915541073466924704, 1.000000000000000000),
 ( 1.000000000000000000, 0.9906898267772793476, 1.000000000000000000),
 ( 1.000000000000000000, 0.9886839553106602230, 1.000000000000000000),
 ( 1.000000000000000000, 0.9875405405517138080, 1.000000000000000000),
 ( 1.000000000000000000, 0.9837407462627784094, 1.000000000000000000),
 ( 1.000000000000000000, 0.9807661871025340483, 1.000000000000000000),
 ( 1.000000000000000000, 0.9740929453405124949, 1.000000000000000000),
 ( 1.000000000000000000, 0.9703914076251105580, 1.000000000000000000),
 ( 1.000000000000000000, 0.9623642252138717712, 1.000000000000000000),
 ( 1.000000000000000000, 0.9580128855153311473, 1.000000000000000000),
 ( 1.000000000000000000, 0.9489407451290137185, 1.000000000000000000),
 ( 1.000000000000000000, 0.9442201479404100928, 1.000000000000000000),
 ( 1.000000000000000000, 0.9345645691926910414, 1.000000000000000000),
 ( 1.000000000000000000, 0.9296290518281515869, 1.000000000000000000),
 ( 1.000000000000000000, 0.9197163133202026497, 1.000000000000000000),
 ( 1.000000000000000000, 0.9147061918368204481, 1.000000000000000000),
 ( 1.000000000000000000, 0.9002701591943753634, 1.000000000000000000),
 ( 1.000000000000000000, 0.8913752732212651964, 1.000000000000000000),
 ( 1.000000000000000000, 0.8822678195319330063, 1.000000000000000000),
 ( 1.000000000000000000, 0.8805477477376374429, 1.000000000000000000),
 ( 1.000000000000000000, 0.8773422126919282471, 1.000000000000000000),
 ( 1.000000000000000000, 0.8758553697949494898, 1.000000000000000000),
 ( 1.000000000000000000, 0.8718595913002757936, 1.000000000000000000),
 ( 1.000000000000000000, 0.8697876269511248815, 1.000000000000000000),
 ( 1.000000000000000000, 0.8669277261913932442, 1.000000000000000000),
 ( 1.000000000000000000, 0.8661397616582809933, 1.000000000000000000),
 ( 1.000000000000000000, 0.8659341656688209765, 1.000000000000000000),
 ( 1.000000000000000000, 0.8665328086759263027, 1.000000000000000000),
 ( 1.000000000000000000, 0.8690449782978997284, 1.000000000000000000),
 ( 1.000000000000000000, 0.8709515724093638278, 1.000000000000000000),
 ( 1.000000000000000000, 0.8746833890562724090, 1.000000000000000000),
 ( 1.000000000000000000, 0.8760725967190144958, 1.000000000000000000),
 ( 1.000000000000000000, 0.8791235325893823616, 1.000000000000000000),
 ( 1.000000000000000000, 0.8807908387558892604, 1.000000000000000000),
 ( 1.000000000000000000, 0.8896941911137391523, 1.000000000000000000),
 ( 1.000000000000000000, 0.8985060072108992379, 1.000000000000000000),
 ( 1.000000000000000000, 0.9128644761645609007, 1.000000000000000000),
 ( 1.000000000000000000, 0.9178532540556407771, 1.000000000000000000),
 ( 1.000000000000000000, 0.9277720463150811447, 1.000000000000000000),
 ( 1.000000000000000000, 0.9327312656600242891, 1.000000000000000000),
 ( 1.000000000000000000, 0.9375990638454466675, 1.000000000000000000) ) ) 
 REPRESENTATION_ITEM ( '' )  SURFACE ( )  );
#17676=EDGE_CURVE ( 'NONE', #5808, #19064, #6052, .T. ) ;
#17714=CARTESIAN_POINT ( 'NONE',  ( 68.09635467782193530, 74.89565063689929048, -3.661860698923952384 ) ) ;
#17740=CARTESIAN_POINT ( 'NONE',  ( 82.80355713680948782, 63.70540732580594323, 0.5609838852837873979 ) ) ;
#17808=CARTESIAN_POINT ( 'NONE',  ( 62.25477568219749003, 78.38020580725381592, -11.99461463175524756 ) ) ;
#17814=CARTESIAN_POINT ( 'NONE',  ( 105.7973891242897650, 30.70991617951901986, -12.50000000000000000 ) ) ;
#17842=CARTESIAN_POINT ( 'NONE',  ( 81.67385617171331091, 66.21413061234055419, 0.6300478184626461253 ) ) ;
#17845=CARTESIAN_POINT ( 'NONE',  ( 75.16299901799432348, 52.17553498020845382, -14.69146284800536684 ) ) ;
#17862=CARTESIAN_POINT ( 'NONE',  ( 77.94818390652243068, 67.33817290270525291, 0.2902393605762963458 ) ) ;
#17883=CARTESIAN_POINT ( 'NONE',  ( 65.28213910571976442, 76.58029512791007676, -19.23060072459815828 ) ) ;
#17919=CARTESIAN_POINT ( 'NONE',  ( 65.40372546169420787, 76.50785360310598548, -5.659300543005241657 ) ) ;
#17933=CARTESIAN_POINT ( 'NONE',  ( 58.65319233816361333, 85.44060140440096518, -13.53501203742773029 ) ) ;
#17944=CARTESIAN_POINT ( 'NONE',  ( 61.96862002106807665, 82.88931969431537539, -6.034168607505590032 ) ) ;
#17946=CARTESIAN_POINT ( 'NONE',  ( 75.56440020197395313, 52.70843083039871857, -8.259164681586764090 ) ) ;
#17947=ORIENTED_EDGE ( 'NONE', *, *, #1409, .T. ) ;
#17959=CARTESIAN_POINT ( 'NONE',  ( 80.91283318083826259, 65.19299774870088982, 0.5000000000000999201 ) ) ;
#17984=CARTESIAN_POINT ( 'NONE',  ( 78.92217576635638920, 67.90907104038892328, -25.20063723745943207 ) ) ;
#18019=CARTESIAN_POINT ( 'NONE',  ( 62.64650668844161885, 78.15169325881764451, -12.59136457139523380 ) ) ;
#18048=CARTESIAN_POINT ( 'NONE',  ( 75.43643680125984474, 52.53826089850589653, -16.21113233865809988 ) ) ;
#18055=ORIENTED_EDGE ( 'NONE', *, *, #17348, .T. ) ;
#18081=CARTESIAN_POINT ( 'NONE',  ( 66.12090498588680987, 76.08041367800895216, -19.94911872569857891 ) ) ;
#18120=CARTESIAN_POINT ( 'NONE',  ( 60.51398719102741097, 84.00985113818899208, -7.546147954418239046 ) ) ;
#18148=CARTESIAN_POINT ( 'NONE',  ( 75.02715018211347342, 51.99577528146775762, -12.09344144936138399 ) ) ;
#18157=CARTESIAN_POINT ( 'NONE',  ( 77.43461555835260413, 55.23580102254843638, -3.894515596738437946 ) ) ;
#18165=CARTESIAN_POINT ( 'NONE',  ( 55.71975233915209458, 77.37356315108866056, -16.50523346184714057 ) ) ;
#18172=CARTESIAN_POINT ( 'NONE',  ( 49.86389338619021316, 127.5895726428436205, -12.50000000000000000 ) ) ;
#18177=CARTESIAN_POINT ( 'NONE',  ( 31.00000000000000711, 65.00000000000000000, -12.50000000000000000 ) ) ;
#18184=CARTESIAN_POINT ( 'NONE',  ( 81.60718771731029619, 62.28998970175522487, -25.21698870735092513 ) ) ;
#18222=CARTESIAN_POINT ( 'NONE',  ( 54.24218927016151781, 78.00150569360116037, -12.67188158619963900 ) ) ;
#18233=AXIS2_PLACEMENT_3D ( 'NONE', #15903, #1274, #19656 ) ;
#18248=CARTESIAN_POINT ( 'NONE',  ( 81.38618934876433286, 61.60889898971228007, 0.05253686650109075373 ) ) ;
#18252=CARTESIAN_POINT ( 'NONE',  ( 78.21123729238362898, 52.55572853022376734, -8.703058536487507268 ) ) ;
#18259=CARTESIAN_POINT ( 'NONE',  ( 81.64154449522867196, 63.92558877093117076, -25.45657102965486018 ) ) ;
#18284=CARTESIAN_POINT ( 'NONE',  ( 81.04710911000414342, 60.81400166747340563, -24.81806225219608208 ) ) ;
#18306=CARTESIAN_POINT ( 'NONE',  ( 81.71672890644845211, 63.56720923707860749, 0.4227506902204759553 ) ) ;
#18331=CARTESIAN_POINT ( 'NONE',  ( 55.32129083036254968, 77.54301705067358341, -15.95188330757220996 ) ) ;
#18347=DIRECTION ( 'NONE',  ( 0.5000000000000041078, -0.8660254037844362651, 0.000000000000000000 ) ) ;
#18368=ORIENTED_EDGE ( 'NONE', *, *, #10790, .T. ) ;
#18369=CARTESIAN_POINT ( 'NONE',  ( 81.06711713768373784, 65.00000000000000000, -25.50000000000000000 ) ) ;
#18396=CARTESIAN_POINT ( 'NONE',  ( 79.48084484536077809, 58.16953689576122599, -23.57162899958074931 ) ) ;
#18433=CARTESIAN_POINT ( 'NONE',  ( 58.64342261736307194, 85.44810595174396894, -13.47428068817142943 ) ) ;
#18434=ADVANCED_FACE ( 'NONE', ( #4885 ), #3389, .T. ) ;
#18458=CARTESIAN_POINT ( 'NONE',  ( 80.19404268355357601, 59.28982122532673316, -0.8110594018112234904 ) ) ;
#18479=EDGE_CURVE ( 'NONE', #5664, #13156, #2010, .T. ) ;
#18497=CARTESIAN_POINT ( 'NONE',  ( 79.54876660668207933, 50.01490354004885575, -15.87845277340799477 ) ) ;
#18503=CARTESIAN_POINT ( 'NONE',  ( 82.91256048669795575, 62.99717322904664485, -25.49106880622069937 ) ) ;
#18522=CARTESIAN_POINT ( 'NONE',  ( 81.71881349453083487, 62.89257827863775674, 0.3300630968703215373 ) ) ;
#18543=CARTESIAN_POINT ( 'NONE',  ( 58.06035037439094282, 76.37624806333415961, -18.80372476195067932 ) ) ;
#18567=CARTESIAN_POINT ( 'NONE',  ( 78.57013627436289482, 56.82968174286880014, -2.376451016691543572 ) ) ;
#18571=CARTESIAN_POINT ( 'NONE',  ( 81.10655718899693056, 54.43739570253208626, -2.927339837274431922 ) ) ;
#18576=CARTESIAN_POINT ( 'NONE',  ( 75.39104360666324567, 52.47794215086291558, -8.991240694413738410 ) ) ;
#18587=LINE ( 'NONE', #15427, #18979 ) ;
#18599=EDGE_CURVE ( 'NONE', #19292, #3901, #1659, .T. ) ;
#18604=CARTESIAN_POINT ( 'NONE',  ( 82.86035624684615186, 61.08028851158093175, -25.16487698176234389 ) ) ;
#18644=CARTESIAN_POINT ( 'NONE',  ( 62.49954260685851892, 78.23754186779291331, -12.52423913820381607 ) ) ;
#18660=DIRECTION ( 'NONE',  ( 1.000000000000000000, -0.000000000000000000, -0.000000000000000000 ) ) ;
#18672=CARTESIAN_POINT ( 'NONE',  ( 79.10968724374433236, 57.61535156440357497, -1.789850051334469283 ) ) ;
#18673=CIRCLE ( 'NONE', #10880, 9.999999999999994671 ) ;
#18733=CARTESIAN_POINT ( 'NONE',  ( 79.44879617809482397, 49.74114623467382046, -10.15578855070954312 ) ) ;
#18748=ORIENTED_EDGE ( 'NONE', *, *, #18479, .F. ) ;
#18777=CARTESIAN_POINT ( 'NONE',  ( 49.86389338619021316, 127.5895726428436205, -12.50000000000000000 ) ) ;
#18779=CARTESIAN_POINT ( 'NONE',  ( 74.42497496061868389, 69.15581319408583738, -0.1672178410544389870 ) ) ;
#18836=CARTESIAN_POINT ( 'NONE',  ( 79.71277097872595618, 50.46579360009113202, -7.932047079679189316 ) ) ;
#18883=CARTESIAN_POINT ( 'NONE',  ( 82.33324130691016762, 62.82700397177379870, 0.3205479543778964602 ) ) ;
#18908=FACE_OUTER_BOUND ( 'NONE', #7121, .T. ) ;
#18923=CARTESIAN_POINT ( 'NONE',  ( 81.06711713768373784, 65.00000000000000000, -25.50000000000000000 ) ) ;
#18932=PRODUCT_DEFINITION_FORMATION_WITH_SPECIFIED_SOURCE ( 'ANY', '', #10402, .NOT_KNOWN. ) ;
#18936=DIRECTION ( 'NONE',  ( 0.000000000000000000, 0.000000000000000000, -1.000000000000000000 ) ) ;
#18947=DIRECTION ( 'NONE',  ( 1.000000000000000000, -0.000000000000000000, -0.000000000000000000 ) ) ;
#18979=VECTOR ( 'NONE', #14260, 1000.000000000000114 ) ;
#18983=DIRECTION ( 'NONE',  ( 0.8660254037844361541, 0.5000000000000044409, 0.000000000000000000 ) ) ;
#18986=CARTESIAN_POINT ( 'NONE',  ( 70.88304643526481641, 70.79367311254448225, -0.8473711193443549394 ) ) ;
#19049=CARTESIAN_POINT ( 'NONE',  ( 79.58732107615884388, 50.12062531598694193, -8.807143433601581251 ) ) ;
#19064=VERTEX_POINT ( 'NONE', #10449 ) ;
#19082=CARTESIAN_POINT ( 'NONE',  ( 67.15136315568796022, 72.45226458839093198, -23.16931136300337357 ) ) ;
#19093=CARTESIAN_POINT ( 'NONE',  ( 82.18628316260415545, 64.02363915056508858, 0.4670741050950639739 ) ) ;
#19138=CARTESIAN_POINT ( 'NONE',  ( 31.00000000000000711, 65.00000000000000000, -25.50000000000000000 ) ) ;
#19152=CIRCLE ( 'NONE', #3227, 4.999999999999998224 ) ;
#19185=CARTESIAN_POINT ( 'NONE',  ( 79.66744006002031142, 66.27074226415487601, -25.44098493566588459 ) ) ;
#19192=CARTESIAN_POINT ( 'NONE',  ( 81.96607779882778289, 65.76354676051263937, 0.6364889541190595912 ) ) ;
#19218=CARTESIAN_POINT ( 'NONE',  ( 82.60162025600570246, 64.43303002238135946, 0.6088031877440995832 ) ) ;
#19280=AXIS2_PLACEMENT_3D ( 'NONE', #957, #18660, #4451 ) ;
#19292=VERTEX_POINT ( 'NONE', #3036 ) ;
#19293=CARTESIAN_POINT ( 'NONE',  ( 58.85476768585063923, 85.28574669046319912, -10.58199671080212489 ) ) ;
#19316=CARTESIAN_POINT ( 'NONE',  ( 81.10655718899290889, 54.43739570252013493, -2.927339837283823520 ) ) ;
#19384=( GEOMETRIC_REPRESENTATION_CONTEXT ( 3 ) GLOBAL_UNCERTAINTY_ASSIGNED_CONTEXT ( ( #5962 ) ) GLOBAL_UNIT_ASSIGNED_CONTEXT ( ( #19886, #17039, #11742 ) ) REPRESENTATION_CONTEXT ( 'NONE', 'WORKASPACE' ) );
#19388=CARTESIAN_POINT ( 'NONE',  ( 63.16228553181007754, 74.18705481243415534, -21.71006526367976974 ) ) ;
#19395=CARTESIAN_POINT ( 'NONE',  ( 61.20179353631819907, 75.03121440969175637, -4.223626890520874255 ) ) ;
#19420=CARTESIAN_POINT ( 'NONE',  ( 79.90495664118901686, 50.99637491787829902, -18.20149439789049239 ) ) ;
#19431=CARTESIAN_POINT ( 'NONE',  ( 78.37318721450539272, 67.09492480576284379, 0.3327101687020665444 ) ) ;
#19449=CARTESIAN_POINT ( 'NONE',  ( 77.32469725096443369, 69.07004555494354747, -24.89440563207301693 ) ) ;
#19485=CARTESIAN_POINT ( 'NONE',  ( 62.17876964677807905, 78.42404429838002500, -11.53082529887307395 ) ) ;
#19491=EDGE_CURVE ( 'NONE', #10603, #6779, #10553, .T. ) ;
#19513=CARTESIAN_POINT ( 'NONE',  ( 60.04195699026302435, 84.37304789033045438, -8.186064125905904376 ) ) ;
#19515=CARTESIAN_POINT ( 'NONE',  ( 78.10850005371658256, 52.36126203026114467, -15.57772792125065919 ) ) ;
#19522=ORIENTED_EDGE ( 'NONE', *, *, #36, .T. ) ;
#19531=CARTESIAN_POINT ( 'NONE',  ( 81.06711713768373784, 65.00000000000000000, 0.4999999999999962252 ) ) ;
#19552=CARTESIAN_POINT ( 'NONE',  ( 67.92197266240974329, 75.00057405452223236, -21.22836514478491665 ) ) ;
#19587=CARTESIAN_POINT ( 'NONE',  ( 62.80918080339837672, 78.05660606650189948, -12.61805735025731146 ) ) ;
#19617=CARTESIAN_POINT ( 'NONE',  ( 60.17750726585534693, 84.26876177917138477, -7.997657589800953204 ) ) ;
#19619=CARTESIAN_POINT ( 'NONE',  ( 79.56530540348451552, 50.06033247906107420, -15.99481843635178535 ) ) ;
#19652=CARTESIAN_POINT ( 'NONE',  ( 76.71035566961047891, 71.19323729334777795, -25.06553181697876909 ) ) ;
#19656=DIRECTION ( 'NONE',  ( 1.000000000000000000, 0.000000000000000000, 0.000000000000000000 ) ) ;
#19660=CARTESIAN_POINT ( 'NONE',  ( 80.43867252173693316, 66.63842558683731454, -25.41598262729068836 ) ) ;
#19696=CARTESIAN_POINT ( 'NONE',  ( 64.30665537872349091, 77.16043010324054308, -6.802757212025057676 ) ) ;
#19697=EDGE_LOOP ( 'NONE', ( #11073, #16201 ) ) ;
#19724=CARTESIAN_POINT ( 'NONE',  ( 75.03434910434744154, 52.00529523017046074, -13.14249383666435200 ) ) ;
#19743=CARTESIAN_POINT ( 'NONE',  ( 64.12703260304576247, 73.76969301591478256, -2.890069931837546680 ) ) ;
#19754=ORIENTED_EDGE ( 'NONE', *, *, #5872, .F. ) ;
#19766=CARTESIAN_POINT ( 'NONE',  ( 81.74095488896709583, 60.03072944676497258, -24.52915917859159123 ) ) ;
#19800=CARTESIAN_POINT ( 'NONE',  ( 62.62356228232910382, 78.16510281290661055, -12.41974233461093569 ) ) ;
#19818=ORIENTED_EDGE ( 'NONE', *, *, #10639, .F. ) ;
#19829=CARTESIAN_POINT ( 'NONE',  ( 79.42243514894403233, 49.66913713435425137, -10.50195963986585568 ) ) ;
#19837=CIRCLE ( 'NONE', #10702, 13.49999999999999645 ) ;
#19843=ORIENTED_EDGE ( 'NONE', *, *, #15499, .F. ) ;
#19866=CARTESIAN_POINT ( 'NONE',  ( 81.45432710247315811, 55.48820219732827752, -22.83971429442600964 ) ) ;
#19886=( LENGTH_UNIT ( ) NAMED_UNIT ( * ) SI_UNIT ( .MILLI., .METRE. ) );
#19909=CARTESIAN_POINT ( 'NONE',  ( 59.05986185621148365, 85.12815607961502451, -15.01156433139877500 ) ) ;
#19932=CARTESIAN_POINT ( 'NONE',  ( 82.29621571355018261, 58.30728878437918183, -0.6895527425001902744 ) ) ;
#19943=CARTESIAN_POINT ( 'NONE',  ( 75.62464799035413421, 52.78861731102380617, -8.028657343369459909 ) ) ;
#19965=CARTESIAN_POINT ( 'NONE',  ( 75.22395539455813207, 72.44174232321687157, -24.78378152481108643 ) ) ;
#19971=CARTESIAN_POINT ( 'NONE',  ( 82.36099222546647525, 65.03795902914596638, -25.63165455292080708 ) ) ;
#19973=CARTESIAN_POINT ( 'NONE',  ( 64.92628429094538944, 80.60227088397526529, -21.04771496906974448 ) ) ;
#19983=CARTESIAN_POINT ( 'NONE',  ( 105.7973891242897508, 30.70991617951901276, -12.50000000000000000 ) ) ;
#19997=CARTESIAN_POINT ( 'NONE',  ( 81.20915916204526752, 64.82231599782905107, 0.5000000000000880407 ) ) ;
#20021=CARTESIAN_POINT ( 'NONE',  ( 56.75722135801910895, 76.93189375612146819, -17.66514001337803919 ) ) ;
#20060=CARTESIAN_POINT ( 'NONE',  ( 81.27728676539042851, 64.71885472535731765, -25.49785049058046837 ) ) ;
#20081=CARTESIAN_POINT ( 'NONE',  ( 80.27267528958725507, 52.02232914097061212, -19.70798756841603350 ) ) ;
#20087=CARTESIAN_POINT ( 'NONE',  ( 82.87350344862416307, 63.33930485192262694, -25.52864195477530984 ) ) ;
#20115=FACE_OUTER_BOUND ( 'NONE', #17555, .T. ) ;
#20122=CARTESIAN_POINT ( 'NONE',  ( 60.93143657513353872, 83.68840998819324284, -17.92058816135999422 ) ) ;
#20156=CARTESIAN_POINT ( 'NONE',  ( 81.45283486207161161, 64.41465532991168175, -25.48770694380405288 ) ) ;
#20169=DIRECTION ( 'NONE',  ( 0.000000000000000000, 0.000000000000000000, 1.000000000000000000 ) ) ;
#20187=DIRECTION ( 'NONE',  ( 0.5000000000000041078, -0.8660254037844361541, 0.000000000000000000 ) ) ;
#20189=CARTESIAN_POINT ( 'NONE',  ( 81.30519808514482349, 55.03237058933864034, -22.52907132704141802 ) ) ;
#20205=CARTESIAN_POINT ( 'NONE',  ( 31.00000000000000711, 65.00000000000000000, -12.50000000000000000 ) ) ;
#20222=CARTESIAN_POINT ( 'NONE',  ( 63.81044076472581850, 77.45544899285202689, -17.65926648166063373 ) ) ;
#20227=CARTESIAN_POINT ( 'NONE',  ( 95.83809698076872507, 24.95991617951895236, -12.50000000000000000 ) ) ;
#20262=CARTESIAN_POINT ( 'NONE',  ( 31.00000000000000711, 75.00000000000000000, -12.50000000000000000 ) ) ;
#20304=DIRECTION ( 'NONE',  ( 1.000000000000000000, -0.000000000000000000, -0.000000000000000000 ) ) ;
#20355=CARTESIAN_POINT ( 'NONE',  ( 81.30365475525482566, 58.89271721487809685, -1.003292558584042649 ) ) ;
#20379=ORIENTED_EDGE ( 'NONE', *, *, #10019, .T. ) ;
#20414=CARTESIAN_POINT ( 'NONE',  ( 79.41606274153808442, 49.65173344286001367, -10.61500173657835155 ) ) ;
#20443=EDGE_LOOP ( 'NONE', ( #18748, #12808 ) ) ;
#20460=CARTESIAN_POINT ( 'NONE',  ( 80.11990493742565889, 66.91023862110843368, 0.3737492815355051845 ) ) ;
#20490=AXIS2_PLACEMENT_3D ( 'NONE', #20262, #13918, #4676 ) ;
#20516=CARTESIAN_POINT ( 'NONE',  ( 86.00000000000000000, 65.00000000000000000, -22.49999999999999645 ) ) ;
#20550=CARTESIAN_POINT ( 'NONE',  ( 75.92249532564342474, 71.86678175105188870, -24.92804124451842540 ) ) ;
#20563=CARTESIAN_POINT ( 'NONE',  ( 75.06454086321275554, 72.57489325992457907, -0.2429554351602942197 ) ) ;
#20596=CARTESIAN_POINT ( 'NONE',  ( 70.73635393167552365, 76.06156464907579107, -23.63261108224246243 ) ) ;
#20615=ORIENTED_EDGE ( 'NONE', *, *, #7916, .T. ) ;
#20617=CARTESIAN_POINT ( 'NONE',  ( 79.78494060632117169, 50.66488423061860402, -7.505244347833114560 ) ) ;
#20665=CARTESIAN_POINT ( 'NONE',  ( 76.76720986645948130, 67.98148330769186032, 0.1575026721056629053 ) ) ;
#20675=CIRCLE ( 'NONE', #15952, 9.999999999999994671 ) ;
#20700=DIRECTION ( 'NONE',  ( 0.000000000000000000, 0.000000000000000000, -1.000000000000000000 ) ) ;
#20748=ORIENTED_EDGE ( 'NONE', *, *, #18479, .T. ) ;
#20763=CARTESIAN_POINT ( 'NONE',  ( 75.60538121466899497, 68.57595208612733018, -25.00629774707486419 ) ) ;
#20770=CARTESIAN_POINT ( 'NONE',  ( 82.31649210851065845, 65.12786813035249622, 0.6330763717910036226 ) ) ;
#20795=CARTESIAN_POINT ( 'NONE',  ( 70.67931723492910123, 76.10686176109747691, -1.383828600441279866 ) ) ;
#20810=ORIENTED_EDGE ( 'NONE', *, *, #3142, .T. ) ;
#20817=AXIS2_PLACEMENT_3D ( 'NONE', #3998, #13756, #10340 ) ;
#20850=VERTEX_POINT ( 'NONE', #10472 ) ;
#20867=CARTESIAN_POINT ( 'NONE',  ( 79.17481878663886619, 68.98945691342343878, 0.4213564493606052896 ) ) ;
#20891=CARTESIAN_POINT ( 'NONE',  ( 82.14226734681926700, 57.73183364759933767, -0.9146047477486081156 ) ) ;
#20916=EDGE_CURVE ( 'NONE', #5375, #14580, #13890, .T. ) ;
#20941=ORIENTED_EDGE ( 'NONE', *, *, #8782, .F. ) ;
#20968=COLOUR_RGB('Light Blue',0.38,0.62,0.78);
#20969=FILL_AREA_STYLE_COLOUR('',#20968);
#20970=FILL_AREA_STYLE('',(#20969));
#20971=SURFACE_STYLE_FILL_AREA(#20970);
#20972=SURFACE_SIDE_STYLE('',(#20971));
#20973=SURFACE_STYLE_USAGE(.BOTH.,#20972);
#20974=PRESENTATION_STYLE_ASSIGNMENT((#20973));
ENDSEC;
END-ISO-10303-21;
